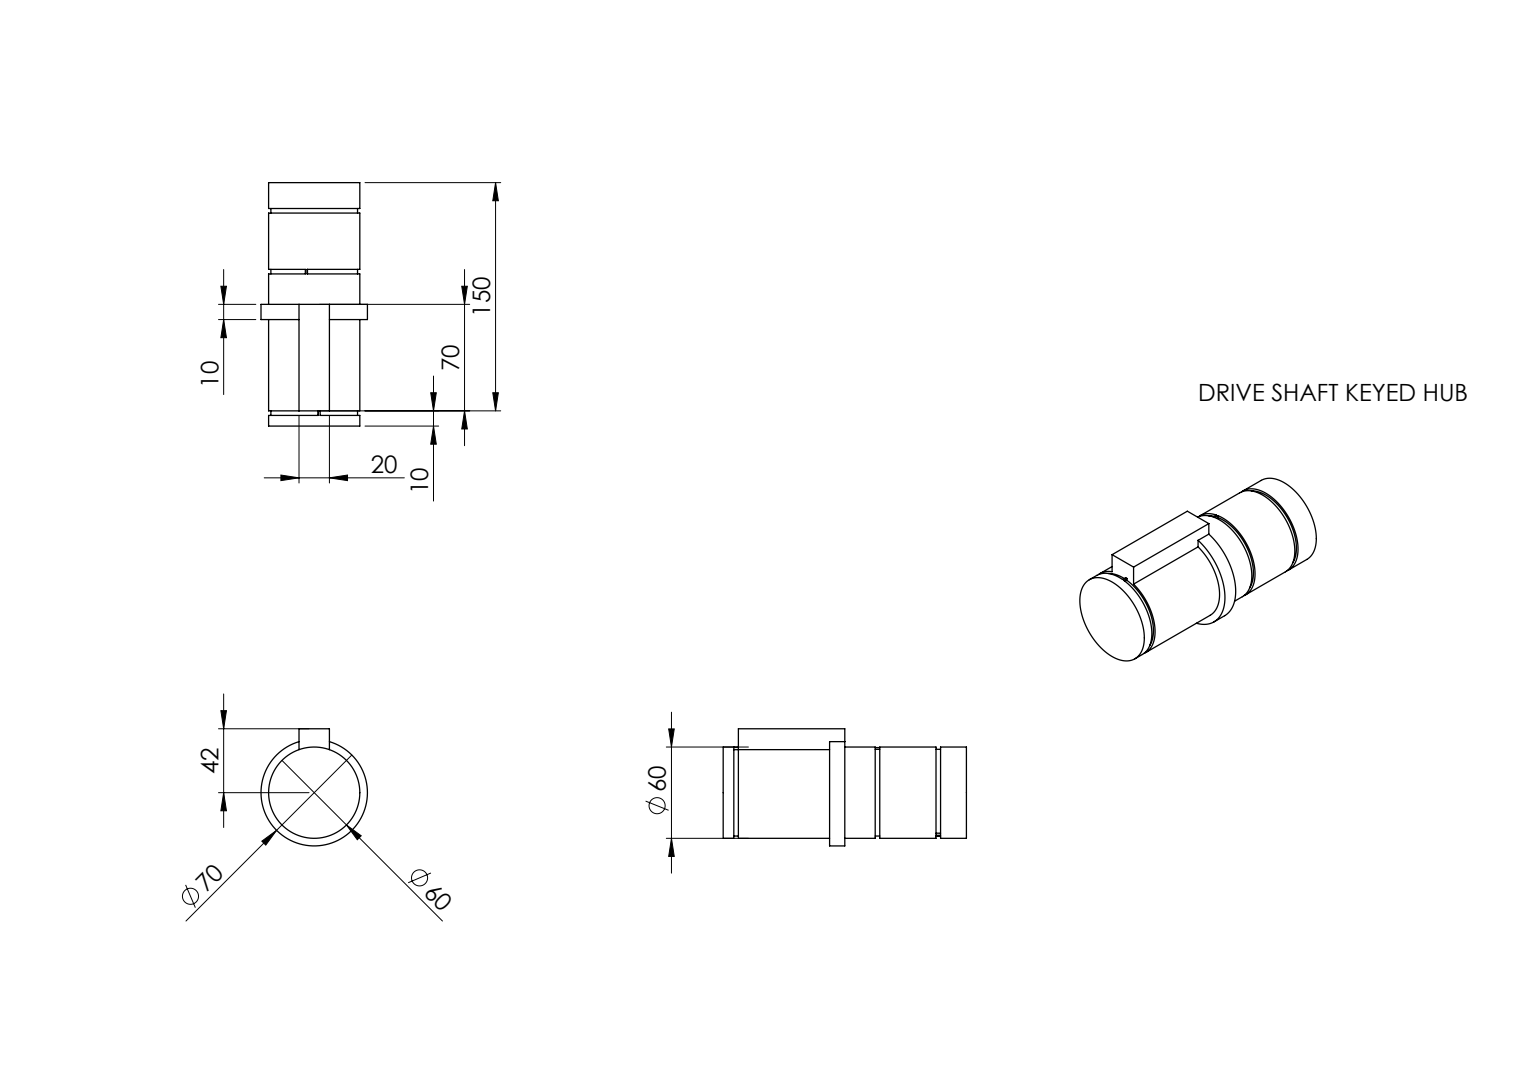
ISO-10303-21;
HEADER;
FILE_DESCRIPTION (('STEP AP214'),
    '1' );
FILE_NAME ('Drive Shaft Keyed Hub.step',
    '2026-10-23T05:12:30',
    ( '' ),
    ( '' ),
    'SwSTEP 2.0',
    'SolidWorks 2026',
    '' );
FILE_SCHEMA (( 'AUTOMOTIVE_DESIGN' ));
ENDSEC;

DATA;
#4=AXIS2_PLACEMENT_3D ( 'NONE', #5314, #2448, #2411 ) ;
#15=ORIENTED_EDGE ( 'NONE', *, *, #7014, .T. ) ;
#22=ORIENTED_EDGE ( 'NONE', *, *, #2120, .F. ) ;
#40=ADVANCED_FACE ( 'NONE', ( #3233 ), #3303, .T. ) ;
#41=ORIENTED_EDGE ( 'NONE', *, *, #4752, .T. ) ;
#44=LINE ( 'NONE', #2388, #7655 ) ;
#46=DIRECTION ( 'NONE',  ( 0.000000000000000000, -1.000000000000000000, 0.000000000000000000 ) ) ;
#47=VERTEX_POINT ( 'NONE', #965 ) ;
#48=EDGE_CURVE ( 'NONE', #5972, #47, #4560, .T. ) ;
#53=DIRECTION ( 'NONE',  ( 0.000000000000000000, 0.000000000000000000, -1.000000000000000000 ) ) ;
#68=LINE ( 'NONE', #4286, #4450 ) ;
#74=CARTESIAN_POINT ( 'NONE',  ( 9.568665290872617746, -28.43309066125681994, -139.9999999999999716 ) ) ;
#84=EDGE_CURVE ( 'NONE', #322, #6002, #3102, .T. ) ;
#89=EDGE_LOOP ( 'NONE', ( #7123, #2974, #1891, #2327 ) ) ;
#90=LINE ( 'NONE', #4231, #2988 ) ;
#97=ORIENTED_EDGE ( 'NONE', *, *, #4752, .F. ) ;
#103=LINE ( 'NONE', #1889, #2646 ) ;
#105=CIRCLE ( 'NONE', #7531, 28.50000000000000355 ) ;
#113=DIRECTION ( 'NONE',  ( 0.9412010056177179118, 0.3378471059875997051, 0.000000000000000000 ) ) ;
#116=ORIENTED_EDGE ( 'NONE', *, *, #4379, .T. ) ;
#118=ORIENTED_EDGE ( 'NONE', *, *, #897, .F. ) ;
#126=EDGE_LOOP ( 'NONE', ( #5453, #5673, #2876, #41 ) ) ;
#131=PRODUCT ( 'Drive Shaft Keyed Hub', 'Drive Shaft Keyed Hub', '', ( #3775 ) ) ;
#134=AXIS2_PLACEMENT_3D ( 'NONE', #2062, #2024, #2612 ) ;
#140=VECTOR ( 'NONE', #2880, 1000.000000000000000 ) ;
#149=ORIENTED_EDGE ( 'NONE', *, *, #2680, .T. ) ;
#150=DIRECTION ( 'NONE',  ( 0.9938725510941108787, -0.1105321318969463978, 0.000000000000000000 ) ) ;
#165=ORIENTED_EDGE ( 'NONE', *, *, #3978, .F. ) ;
#178=LINE ( 'NONE', #6692, #6392 ) ;
#180=STYLED_ITEM ( 'NONE', ( #6391 ), #5011 ) ;
#181=ADVANCED_FACE ( 'NONE', ( #7711 ), #4121, .F. ) ;
#188=ORIENTED_EDGE ( 'NONE', *, *, #6602, .F. ) ;
#194=VERTEX_POINT ( 'NONE', #3652 ) ;
#197=CARTESIAN_POINT ( 'NONE',  ( -5.554394503829287011, 27.95350964898380752, -79.99999999999995737 ) ) ;
#200=EDGE_LOOP ( 'NONE', ( #6714, #643, #5819, #2337 ) ) ;
#203=CARTESIAN_POINT ( 'NONE',  ( 9.090232026328989079, -27.01143612819398143, -119.9999999999999716 ) ) ;
#205=CARTESIAN_POINT ( 'NONE',  ( 9.090232026328989079, -27.01143612819398143, -122.9999999999999716 ) ) ;
#207=AXIS2_PLACEMENT_3D ( 'NONE', #2317, #4702, #7112 ) ;
#214=CARTESIAN_POINT ( 'NONE',  ( 5.777789833161707559E-31, -4.119912841284263785E-15, -119.9999999999999716 ) ) ;
#224=DIRECTION ( 'NONE',  ( 0.000000000000000000, 0.000000000000000000, -1.000000000000000000 ) ) ;
#226=CARTESIAN_POINT ( 'NONE',  ( -28.05900627794857627, -4.994213320838723824, -79.99999999999995737 ) ) ;
#228=DIRECTION ( 'NONE',  ( 0.000000000000000000, 0.000000000000000000, -1.000000000000000000 ) ) ;
#247=DIRECTION ( 'NONE',  ( -1.000000000000000000, 0.000000000000000000, 0.000000000000000000 ) ) ;
#249=DIRECTION ( 'NONE',  ( -0.09063257223759993431, -0.9958843993404034034, 0.000000000000000000 ) ) ;
#252=CYLINDRICAL_SURFACE ( 'NONE', #6988, 29.99999999999999289 ) ;
#256=VERTEX_POINT ( 'NONE', #1883 ) ;
#259=DIRECTION ( 'NONE',  ( -0.000000000000000000, -0.000000000000000000, 1.000000000000000000 ) ) ;
#264=ORIENTED_EDGE ( 'NONE', *, *, #3362, .F. ) ;
#266=ORIENTED_EDGE ( 'NONE', *, *, #6459, .F. ) ;
#267=CARTESIAN_POINT ( 'NONE',  ( 0.000000000000000000, 0.000000000000000000, -139.9999999999999716 ) ) ;
#270=CARTESIAN_POINT ( 'NONE',  ( 10.00000000000000000, 41.99999999999999289, -60.00000000000000711 ) ) ;
#279=FACE_OUTER_BOUND ( 'NONE', #4266, .T. ) ;
#281=ORIENTED_EDGE ( 'NONE', *, *, #3745, .T. ) ;
#284=CARTESIAN_POINT ( 'NONE',  ( 0.000000000000000000, 0.000000000000000000, -122.9999999999999716 ) ) ;
#287=CARTESIAN_POINT ( 'NONE',  ( 0.000000000000000000, 0.000000000000000000, -60.00000000000000000 ) ) ;
#292=EDGE_LOOP ( 'NONE', ( #3015, #4779, #3543, #2009 ) ) ;
#299=CARTESIAN_POINT ( 'NONE',  ( -10.00000000000000000, 28.28427124746189136, -50.00000000000000000 ) ) ;
#301=DIRECTION ( 'NONE',  ( 0.9412010056177179118, 0.3378471059875997051, 0.000000000000000000 ) ) ;
#303=VECTOR ( 'NONE', #4360, 1000.000000000000000 ) ;
#304=ORIENTED_EDGE ( 'NONE', *, *, #4363, .T. ) ;
#319=CIRCLE ( 'NONE', #5110, 29.99999999999999289 ) ;
#322=VERTEX_POINT ( 'NONE', #3771 ) ;
#333=ORIENTED_EDGE ( 'NONE', *, *, #3563, .F. ) ;
#341=CIRCLE ( 'NONE', #4254, 29.99999999999999289 ) ;
#344=ORIENTED_EDGE ( 'NONE', *, *, #1290, .F. ) ;
#349=CARTESIAN_POINT ( 'NONE',  ( 28.05900627794855851, 4.994213320838720271, -82.99999999999995737 ) ) ;
#353=CIRCLE ( 'NONE', #4261, 29.99999999999999289 ) ;
#368=DIRECTION ( 'NONE',  ( -1.000000000000000000, 0.000000000000000000, 0.000000000000000000 ) ) ;
#369=EDGE_CURVE ( 'NONE', #2537, #7447, #319, .T. ) ;
#382=AXIS2_PLACEMENT_3D ( 'NONE', #2843, #7643, #5876 ) ;
#383=ORIENTED_EDGE ( 'NONE', *, *, #6065, .F. ) ;
#385=DIRECTION ( 'NONE',  ( -1.000000000000000000, 0.000000000000000000, 0.000000000000000000 ) ) ;
#387=VERTEX_POINT ( 'NONE', #5026 ) ;
#394=EDGE_CURVE ( 'NONE', #2888, #7603, #5583, .T. ) ;
#398=DIRECTION ( 'NONE',  ( 1.000000000000000000, 0.000000000000000000, 0.000000000000000000 ) ) ;
#400=EDGE_CURVE ( 'NONE', #6073, #6532, #1763, .T. ) ;
#415=AXIS2_PLACEMENT_3D ( 'NONE', #6467, #428, #4730 ) ;
#427=FILL_AREA_STYLE ('',( #1657 ) ) ;
#428=DIRECTION ( 'NONE',  ( 3.081487911019577365E-33, -2.775557561562891967E-17, -1.000000000000000000 ) ) ;
#442=DIRECTION ( 'NONE',  ( 0.000000000000000000, 0.000000000000000000, 1.000000000000000000 ) ) ;
#443=DIRECTION ( 'NONE',  ( 1.000000000000000000, 0.000000000000000000, -0.000000000000000000 ) ) ;
#452=AXIS2_PLACEMENT_3D ( 'NONE', #5129, #1347, #6245 ) ;
#458=CARTESIAN_POINT ( 'NONE',  ( -6.873268260756527152E-15, 0.000000000000000000, -79.99999999999995737 ) ) ;
#459=ADVANCED_FACE ( 'NONE', ( #3218 ), #2157, .T. ) ;
#464=ORIENTED_EDGE ( 'NONE', *, *, #7412, .F. ) ;
#479=CARTESIAN_POINT ( 'NONE',  ( -7.039801714450301422E-15, 0.000000000000000000, -82.99999999999995737 ) ) ;
#480=AXIS2_PLACEMENT_3D ( 'NONE', #5844, #4103, #2188 ) ;
#481=DIRECTION ( 'NONE',  ( -0.000000000000000000, -0.000000000000000000, -1.000000000000000000 ) ) ;
#484=AXIS2_PLACEMENT_3D ( 'NONE', #5502, #2370, #2407 ) ;
#489=AXIS2_PLACEMENT_3D ( 'NONE', #1675, #1035, #3446 ) ;
#494=AXIS2_PLACEMENT_3D ( 'NONE', #1361, #3659, #3110 ) ;
#503=ORIENTED_EDGE ( 'NONE', *, *, #3907, .F. ) ;
#507=SURFACE_STYLE_FILL_AREA ( #427 ) ;
#512=EDGE_CURVE ( 'NONE', #3634, #5216, #2318, .T. ) ;
#518=CARTESIAN_POINT ( 'NONE',  ( 29.99999999999999289, 0.000000000000000000, -139.9999999999999716 ) ) ;
#526=FACE_OUTER_BOUND ( 'NONE', #5662, .T. ) ;
#531=VECTOR ( 'NONE', #6993, 1000.000000000000114 ) ;
#538=CYLINDRICAL_SURFACE ( 'NONE', #6515, 28.50000000000000711 ) ;
#542=AXIS2_PLACEMENT_3D ( 'NONE', #7456, #6279, #2065 ) ;
#558=EDGE_CURVE ( 'NONE', #1483, #3701, #583, .T. ) ;
#559=CARTESIAN_POINT ( 'NONE',  ( -10.00000000000000000, 28.28427124746189136, 10.00000000000000000 ) ) ;
#573=EDGE_CURVE ( 'NONE', #6864, #6819, #3734, .T. ) ;
#578=VERTEX_POINT ( 'NONE', #6013 ) ;
#583=CIRCLE ( 'NONE', #702, 29.99999999999999289 ) ;
#587=VERTEX_POINT ( 'NONE', #644 ) ;
#596=CARTESIAN_POINT ( 'NONE',  ( 0.000000000000000000, 0.000000000000000000, -79.99999999999995737 ) ) ;
#597=CYLINDRICAL_SURFACE ( 'NONE', #4258, 29.99999999999999289 ) ;
#599=VERTEX_POINT ( 'NONE', #3056 ) ;
#600=VECTOR ( 'NONE', #7039, 1000.000000000000000 ) ;
#613=ORIENTED_EDGE ( 'NONE', *, *, #2264, .T. ) ;
#617=AXIS2_PLACEMENT_3D ( 'NONE', #4825, #53, #3645 ) ;
#626=ORIENTED_EDGE ( 'NONE', *, *, #707, .F. ) ;
#628=ORIENTED_EDGE ( 'NONE', *, *, #2216, .T. ) ;
#629=CARTESIAN_POINT ( 'NONE',  ( -1.728922298134113098E-15, 8.513302795252935035E-16, 10.00000000000000000 ) ) ;
#635=ORIENTED_EDGE ( 'NONE', *, *, #878, .T. ) ;
#636=AXIS2_PLACEMENT_3D ( 'NONE', #596, #7064, #5883 ) ;
#643=ORIENTED_EDGE ( 'NONE', *, *, #5237, .F. ) ;
#644=CARTESIAN_POINT ( 'NONE',  ( 29.99999999999999289, 0.000000000000000000, -60.00000000000000000 ) ) ;
#667=LINE ( 'NONE', #5442, #3443 ) ;
#672=EDGE_CURVE ( 'NONE', #3192, #3615, #90, .T. ) ;
#681=VECTOR ( 'NONE', #5176, 1000.000000000000000 ) ;
#682=CARTESIAN_POINT ( 'NONE',  ( 3.716043017018883621, 28.25669875083898930, 13.00000000000000178 ) ) ;
#683=CARTESIAN_POINT ( 'NONE',  ( -26.82422866010495710, -9.628642520646591763, -122.9999999999999716 ) ) ;
#692=DIRECTION ( 'NONE',  ( 0.000000000000000000, 0.000000000000000000, 1.000000000000000000 ) ) ;
#700=ADVANCED_FACE ( 'NONE', ( #3679 ), #2979, .T. ) ;
#702=AXIS2_PLACEMENT_3D ( 'NONE', #2238, #7036, #2274 ) ;
#706=DIRECTION ( 'NONE',  ( -0.000000000000000000, 1.000000000000000000, 0.000000000000000000 ) ) ;
#707=EDGE_CURVE ( 'NONE', #2049, #6833, #1270, .T. ) ;
#709=CIRCLE ( 'NONE', #6257, 28.50000000000000711 ) ;
#711=CYLINDRICAL_SURFACE ( 'NONE', #6817, 29.99999999999999289 ) ;
#726=ORIENTED_EDGE ( 'NONE', *, *, #6984, .F. ) ;
#750=DIRECTION ( 'NONE',  ( 0.000000000000000000, 0.000000000000000000, 1.000000000000000000 ) ) ;
#751=FACE_OUTER_BOUND ( 'NONE', #3367, .T. ) ;
#757=EDGE_CURVE ( 'NONE', #3192, #1710, #4102, .T. ) ;
#770=DIRECTION ( 'NONE',  ( -0.1555099737793451398, 0.9878343221690302212, -1.110223024625155986E-18 ) ) ;
#775=EDGE_LOOP ( 'NONE', ( #5683, #7161, #971, #2534, #5294, #5753, #1571, #266 ) ) ;
#778=CARTESIAN_POINT ( 'NONE',  ( -7.039801714450301422E-15, 0.000000000000000000, -82.99999999999995737 ) ) ;
#779=AXIS2_PLACEMENT_3D ( 'NONE', #837, #6286, #2075 ) ;
#783=PRODUCT_DEFINITION_FORMATION_WITH_SPECIFIED_SOURCE ( 'ANY', '', #131, .NOT_KNOWN. ) ;
#792=VECTOR ( 'NONE', #1139, 1000.000000000000000 ) ;
#804=FACE_OUTER_BOUND ( 'NONE', #126, .T. ) ;
#811=ORIENTED_EDGE ( 'NONE', *, *, #4867, .T. ) ;
#823=AXIS2_PLACEMENT_3D ( 'NONE', #1004, #3418, #6495 ) ;
#837=CARTESIAN_POINT ( 'NONE',  ( -1.728922298134113098E-15, 8.513302795252935035E-16, 13.00000000000000178 ) ) ;
#841=DIRECTION ( 'NONE',  ( 0.000000000000000000, -1.000000000000000000, 0.000000000000000000 ) ) ;
#842=VECTOR ( 'NONE', #3621, 1000.000000000000000 ) ;
#845=DIRECTION ( 'NONE',  ( -0.000000000000000000, -0.000000000000000000, 1.000000000000000000 ) ) ;
#859=VECTOR ( 'NONE', #5866, 1000.000000000000000 ) ;
#861=DIRECTION ( 'NONE',  ( 1.000000000000000000, 0.000000000000000000, -0.000000000000000000 ) ) ;
#865=CARTESIAN_POINT ( 'NONE',  ( -6.873268260756527152E-15, 0.000000000000000000, -79.99999999999995737 ) ) ;
#866=DIRECTION ( 'NONE',  ( 0.000000000000000000, 0.000000000000000000, -1.000000000000000000 ) ) ;
#876=CARTESIAN_POINT ( 'NONE',  ( 0.000000000000000000, 0.000000000000000000, -50.00000000000000000 ) ) ;
#878=EDGE_CURVE ( 'NONE', #5239, #4532, #709, .T. ) ;
#882=DIRECTION ( 'NONE',  ( 0.000000000000000000, 0.000000000000000000, 1.000000000000000000 ) ) ;
#883=AXIS2_PLACEMENT_3D ( 'NONE', #1655, #1745, #6464 ) ;
#886=VERTEX_POINT ( 'NONE', #1504 ) ;
#897=EDGE_CURVE ( 'NONE', #5940, #2183, #5745, .T. ) ;
#911=VECTOR ( 'NONE', #4475, 1000.000000000000000 ) ;
#915=CARTESIAN_POINT ( 'NONE',  ( 28.05900627794856206, 4.994213320838721160, -79.99999999999995737 ) ) ;
#916=AXIS2_PLACEMENT_3D ( 'NONE', #6341, #927, #3343 ) ;
#921=DIRECTION ( 'NONE',  ( 3.081487911019577365E-33, -2.775557561562891967E-17, -1.000000000000000000 ) ) ;
#927=DIRECTION ( 'NONE',  ( 0.000000000000000000, 0.000000000000000000, 1.000000000000000000 ) ) ;
#928=VECTOR ( 'NONE', #3765, 1000.000000000000114 ) ;
#929=DIRECTION ( 'NONE',  ( 0.3566035499204626702, -0.9342558044690565389, 2.649161120199466423E-17 ) ) ;
#939=CARTESIAN_POINT ( 'NONE',  ( 29.99999999999999289, 0.000000000000000000, -139.9999999999999716 ) ) ;
#948=CARTESIAN_POINT ( 'NONE',  ( -29.99999999999999289, 3.673940397442058389E-15, -122.9999999999999716 ) ) ;
#950=CARTESIAN_POINT ( 'NONE',  ( -4.665299213380365018, 29.63502966507090619, -139.9999999999999716 ) ) ;
#952=VERTEX_POINT ( 'NONE', #1020 ) ;
#960=DIRECTION ( 'NONE',  ( 5.551115123125782702E-17, 0.000000000000000000, 1.000000000000000000 ) ) ;
#965=CARTESIAN_POINT ( 'NONE',  ( -4.432034252711344102, 28.15327818181735964, -82.99999999999995737 ) ) ;
#971=ORIENTED_EDGE ( 'NONE', *, *, #5971, .T. ) ;
#972=ORIENTED_EDGE ( 'NONE', *, *, #2975, .F. ) ;
#973=ORIENTED_EDGE ( 'NONE', *, *, #1738, .F. ) ;
#981=AXIS2_PLACEMENT_3D ( 'NONE', #197, #6831, #1415 ) ;
#1003=EDGE_CURVE ( 'NONE', #3123, #7368, #6511, .T. ) ;
#1004=CARTESIAN_POINT ( 'NONE',  ( -1.728922298134113098E-15, 8.513302795252935035E-16, 13.00000000000000178 ) ) ;
#1008=CIRCLE ( 'NONE', #134, 29.99999999999999289 ) ;
#1013=AXIS2_PLACEMENT_3D ( 'NONE', #629, #4330, #150 ) ;
#1016=( NAMED_UNIT ( * ) PLANE_ANGLE_UNIT ( ) SI_UNIT ( $, .RADIAN. ) );
#1020=CARTESIAN_POINT ( 'NONE',  ( -5.554394503829287011, 27.95350964898380752, -79.99999999999995737 ) ) ;
#1027=EDGE_CURVE ( 'NONE', #5335, #5921, #6769, .T. ) ;
#1030=ADVANCED_FACE ( 'NONE', ( #7613 ), #2230, .F. ) ;
#1035=DIRECTION ( 'NONE',  ( 0.9958843993404035144, -0.09063257223759993431, 0.000000000000000000 ) ) ;
#1039=CARTESIAN_POINT ( 'NONE',  ( -4.432034252711344102, 28.15327818181735964, -79.99999999999995737 ) ) ;
#1043=VERTEX_POINT ( 'NONE', #5371 ) ;
#1044=ADVANCED_FACE ( 'NONE', ( #1431 ), #3848, .F. ) ;
#1047=DIRECTION ( 'NONE',  ( -3.081487911019577365E-33, 2.775557561562891967E-17, 1.000000000000000000 ) ) ;
#1049=VECTOR ( 'NONE', #6193, 1000.000000000000000 ) ;
#1051=VERTEX_POINT ( 'NONE', #6214 ) ;
#1057=CARTESIAN_POINT ( 'NONE',  ( 10.16320117273318679, -26.62629042736811869, -122.9999999999999716 ) ) ;
#1059=SURFACE_SIDE_STYLE ('',( #507 ) ) ;
#1061=AXIS2_PLACEMENT_3D ( 'NONE', #6484, #7155, #7343 ) ;
#1076=CARTESIAN_POINT ( 'NONE',  ( -10.00000000000000000, 0.000000000000000000, -60.00000000000000711 ) ) ;
#1084=EDGE_CURVE ( 'NONE', #2183, #6897, #6251, .T. ) ;
#1098=CIRCLE ( 'NONE', #5510, 29.99999999999999289 ) ;
#1102=VERTEX_POINT ( 'NONE', #6177 ) ;
#1105=DIRECTION ( 'NONE',  ( 0.9412010056177179118, 0.3378471059875997051, 0.000000000000000000 ) ) ;
#1106=CARTESIAN_POINT ( 'NONE',  ( -6.873268260756527152E-15, 0.000000000000000000, -79.99999999999995737 ) ) ;
#1108=CARTESIAN_POINT ( 'NONE',  ( -29.99999999999999289, 3.673940397442058389E-15, 10.00000000000000888 ) ) ;
#1119=CARTESIAN_POINT ( 'NONE',  ( -28.05900627794857272, -4.994213320838722936, -79.99999999999995737 ) ) ;
#1124=CARTESIAN_POINT ( 'NONE',  ( -7.039801714450301422E-15, 0.000000000000000000, -82.99999999999995737 ) ) ;
#1126=LINE ( 'NONE', #4642, #3627 ) ;
#1134=AXIS2_PLACEMENT_3D ( 'NONE', #4260, #7227, #1827 ) ;
#1139=DIRECTION ( 'NONE',  ( -0.1555099737793451675, 0.9878343221690302212, -1.110223024625155986E-18 ) ) ;
#1140=EDGE_CURVE ( 'NONE', #4191, #4160, #4986, .T. ) ;
#1146=DIRECTION ( 'NONE',  ( 0.9845265360683707057, 0.1752355551171480841, 0.000000000000000000 ) ) ;
#1147=DIRECTION ( 'NONE',  ( 0.000000000000000000, 0.000000000000000000, 1.000000000000000000 ) ) ;
#1162=CIRCLE ( 'NONE', #3063, 29.99999999999999289 ) ;
#1173=EDGE_LOOP ( 'NONE', ( #97, #3739, #149, #5750, #3439, #1470 ) ) ;
#1179=MECHANICAL_DESIGN_GEOMETRIC_PRESENTATION_REPRESENTATION('',(#3832),#5212);
#1199=LINE ( 'NONE', #4350, #6780 ) ;
#1205=LINE ( 'NONE', #3620, #3011 ) ;
#1206=DIRECTION ( 'NONE',  ( 0.000000000000000000, 0.000000000000000000, -1.000000000000000000 ) ) ;
#1217=LINE ( 'NONE', #4845, #1423 ) ;
#1224=FACE_OUTER_BOUND ( 'NONE', #5370, .T. ) ;
#1232=CARTESIAN_POINT ( 'NONE',  ( 0.000000000000000000, 0.000000000000000000, -139.9999999999999716 ) ) ;
#1248=CARTESIAN_POINT ( 'NONE',  ( 10.00000000000000000, 28.28427124746189136, 10.00000000000000888 ) ) ;
#1258=CARTESIAN_POINT ( 'NONE',  ( -29.99999999999999289, 3.673940397442058389E-15, 13.00000000000001066 ) ) ;
#1267=ORIENTED_EDGE ( 'NONE', *, *, #5379, .T. ) ;
#1270=LINE ( 'NONE', #682, #7760 ) ;
#1282=LINE ( 'NONE', #3774, #4249 ) ;
#1287=ORIENTED_EDGE ( 'NONE', *, *, #1958, .T. ) ;
#1290=EDGE_CURVE ( 'NONE', #6532, #7160, #3619, .T. ) ;
#1300=DIRECTION ( 'NONE',  ( 1.000000000000000000, 0.000000000000000000, 0.000000000000000000 ) ) ;
#1301=CARTESIAN_POINT ( 'NONE',  ( 0.000000000000000000, 0.000000000000000000, 0.000000000000000000 ) ) ;
#1306=ORIENTED_EDGE ( 'NONE', *, *, #5427, .F. ) ;
#1310=DIRECTION ( 'NONE',  ( -1.000000000000000000, -8.881784197001252323E-16, 0.000000000000000000 ) ) ;
#1315=AXIS2_PLACEMENT_3D ( 'NONE', #7626, #4670, #6374 ) ;
#1318=DIRECTION ( 'NONE',  ( 0.1303874742813643239, 0.9914631140645255858, 0.000000000000000000 ) ) ;
#1324=DIRECTION ( 'NONE',  ( 0.000000000000000000, 0.000000000000000000, -1.000000000000000000 ) ) ;
#1325=VERTEX_POINT ( 'NONE', #3442 ) ;
#1331=DIRECTION ( 'NONE',  ( 3.081487911019577365E-33, -2.775557561562891967E-17, -1.000000000000000000 ) ) ;
#1332=CYLINDRICAL_SURFACE ( 'NONE', #6222, 28.50000000000000711 ) ;
#1346=ORIENTED_EDGE ( 'NONE', *, *, #4608, .F. ) ;
#1347=DIRECTION ( 'NONE',  ( 5.551115123125782702E-17, -0.000000000000000000, 1.000000000000000000 ) ) ;
#1357=DIRECTION ( 'NONE',  ( -0.000000000000000000, -0.000000000000000000, 1.000000000000000000 ) ) ;
#1361=CARTESIAN_POINT ( 'NONE',  ( 0.000000000000000000, 0.000000000000000000, -60.00000000000000711 ) ) ;
#1362=ORIENTED_EDGE ( 'NONE', *, *, #1084, .F. ) ;
#1363=EDGE_LOOP ( 'NONE', ( #383, #2492 ) ) ;
#1368=CARTESIAN_POINT ( 'NONE',  ( 5.870234470492294880E-31, -4.203179568131150526E-15, -122.9999999999999716 ) ) ;
#1371=ORIENTED_EDGE ( 'NONE', *, *, #1525, .F. ) ;
#1377=EDGE_CURVE ( 'NONE', #1051, #6864, #5904, .T. ) ;
#1382=CARTESIAN_POINT ( 'NONE',  ( 3.911624228440929052, 29.74389342193576624, 13.00000000000001066 ) ) ;
#1383=ORIENTED_EDGE ( 'NONE', *, *, #3503, .F. ) ;
#1387=PRODUCT_DEFINITION_SHAPE ( 'NONE', 'NONE',  #6478 ) ;
#1392=LINE ( 'NONE', #205, #6581 ) ;
#1393=ORIENTED_EDGE ( 'NONE', *, *, #6504, .T. ) ;
#1409=EDGE_LOOP ( 'NONE', ( #1796, #3155, #6670, #4098, #6477, #628 ) ) ;
#1413=DIRECTION ( 'NONE',  ( 0.9845265360683707057, 0.1752355551171480841, 0.000000000000000000 ) ) ;
#1415=DIRECTION ( 'NONE',  ( 0.1948910352220799835, -0.9808248999643441879, -1.110223024625155986E-18 ) ) ;
#1423=VECTOR ( 'NONE', #706, 1000.000000000000000 ) ;
#1431=FACE_OUTER_BOUND ( 'NONE', #2465, .T. ) ;
#1443=EDGE_CURVE ( 'NONE', #7492, #5665, #1126, .T. ) ;
#1446=CLOSED_SHELL ( 'NONE', ( #6737, #6352, #1475, #5330, #3466, #2829, #4656, #459, #3800, #2519, #2309, #7588, #4374, #5871, #7324, #3599, #2557, #7263, #7513, #700, #4765, #1030, #2895, #40, #4909, #3685, #2653, #2637, #1589, #5674, #181, #5443, #6790, #5617, #2777, #1044, #5963, #4858, #7757, #1575 ) ) ;
#1465=AXIS2_PLACEMENT_3D ( 'NONE', #1909, #5531, #2395 ) ;
#1470=ORIENTED_EDGE ( 'NONE', *, *, #7693, .T. ) ;
#1475=ADVANCED_FACE ( 'NONE', ( #3538 ), #538, .T. ) ;
#1481=DIRECTION ( 'NONE',  ( 3.081487911019577365E-33, -2.775557561562891967E-17, -1.000000000000000000 ) ) ;
#1482=EDGE_LOOP ( 'NONE', ( #6953, #7658, #5675, #1661, #7308, #6188, #4056, #2700 ) ) ;
#1483=VERTEX_POINT ( 'NONE', #2371 ) ;
#1486=EDGE_CURVE ( 'NONE', #7492, #2049, #3874, .T. ) ;
#1495=ORIENTED_EDGE ( 'NONE', *, *, #7454, .F. ) ;
#1497=DIRECTION ( 'NONE',  ( 0.000000000000000000, 0.000000000000000000, 1.000000000000000000 ) ) ;
#1504=CARTESIAN_POINT ( 'NONE',  ( -28.32536770618215982, 3.150165759062969695, 10.00000000000000000 ) ) ;
#1505=CARTESIAN_POINT ( 'NONE',  ( 28.32536770618215982, -3.150165759062971471, 13.00000000000000178 ) ) ;
#1507=AXIS2_PLACEMENT_3D ( 'NONE', #6309, #7594, #7009 ) ;
#1511=AXIS2_PLACEMENT_3D ( 'NONE', #5290, #6517, #6472 ) ;
#1519=VECTOR ( 'NONE', #1931, 1000.000000000000000 ) ;
#1521=ORIENTED_EDGE ( 'NONE', *, *, #7357, .F. ) ;
#1522=EDGE_CURVE ( 'NONE', #2129, #7160, #1282, .T. ) ;
#1525=EDGE_CURVE ( 'NONE', #4724, #194, #4873, .T. ) ;
#1545=DIRECTION ( 'NONE',  ( 1.000000000000000000, 0.000000000000000000, 0.000000000000000000 ) ) ;
#1552=CARTESIAN_POINT ( 'NONE',  ( -4.665299213380359689, 29.63502966507089909, -79.99999999999995737 ) ) ;
#1553=PLANE ( 'NONE',  #489 ) ;
#1559=VECTOR ( 'NONE', #6445, 1000.000000000000000 ) ;
#1562=DIRECTION ( 'NONE',  ( -5.551115123125782702E-17, 0.000000000000000000, -1.000000000000000000 ) ) ;
#1564=COLOUR_RGB ( '',0.8941176470588234615, 0.8941176470588234615, 0.8941176470588234615 ) ;
#1571=ORIENTED_EDGE ( 'NONE', *, *, #5379, .F. ) ;
#1573=VERTEX_POINT ( 'NONE', #4989 ) ;
#1575=ADVANCED_FACE ( 'NONE', ( #4243 ), #3067, .T. ) ;
#1588=LINE ( 'NONE', #5293, #531 ) ;
#1589=ADVANCED_FACE ( 'NONE', ( #4357 ), #3691, .F. ) ;
#1591=AXIS2_PLACEMENT_3D ( 'NONE', #7063, #5328, #7728 ) ;
#1596=CARTESIAN_POINT ( 'NONE',  ( 29.99999999999999289, 0.000000000000000000, -139.9999999999999716 ) ) ;
#1601=VERTEX_POINT ( 'NONE', #2597 ) ;
#1616=DIRECTION ( 'NONE',  ( 0.000000000000000000, 0.000000000000000000, 1.000000000000000000 ) ) ;
#1619=EDGE_CURVE ( 'NONE', #3881, #2383, #178, .T. ) ;
#1627=ORIENTED_EDGE ( 'NONE', *, *, #5133, .F. ) ;
#1635=FACE_OUTER_BOUND ( 'NONE', #3761, .T. ) ;
#1654=AXIS2_PLACEMENT_3D ( 'NONE', #1124, #2331, #5941 ) ;
#1655=CARTESIAN_POINT ( 'NONE',  ( -1.728922298134113098E-15, 8.513302795252935035E-16, 13.00000000000000178 ) ) ;
#1657=FILL_AREA_STYLE_COLOUR ( '', #1564 ) ;
#1658=FACE_OUTER_BOUND ( 'NONE', #6506, .T. ) ;
#1661=ORIENTED_EDGE ( 'NONE', *, *, #5964, .T. ) ;
#1672=CIRCLE ( 'NONE', #5195, 29.99999999999999289 ) ;
#1675=CARTESIAN_POINT ( 'NONE',  ( 2.583028308771596837, 28.38270538120150377, 13.00000000000000178 ) ) ;
#1679=ORIENTED_EDGE ( 'NONE', *, *, #2459, .F. ) ;
#1689=CARTESIAN_POINT ( 'NONE',  ( 26.82422866010495710, 9.628642520646586433, -119.9999999999999716 ) ) ;
#1691=EDGE_CURVE ( 'NONE', #6167, #587, #1098, .T. ) ;
#1693=EDGE_LOOP ( 'NONE', ( #1306, #6106, #1845, #1679, #5241, #2719 ) ) ;
#1710=VERTEX_POINT ( 'NONE', #2668 ) ;
#1716=DIRECTION ( 'NONE',  ( 1.000000000000000000, 0.000000000000000000, 0.000000000000000000 ) ) ;
#1727=EDGE_CURVE ( 'NONE', #194, #5633, #2123, .T. ) ;
#1738=EDGE_CURVE ( 'NONE', #1573, #322, #3257, .T. ) ;
#1745=DIRECTION ( 'NONE',  ( 0.000000000000000000, 0.000000000000000000, 1.000000000000000000 ) ) ;
#1754=CYLINDRICAL_SURFACE ( 'NONE', #5016, 29.99999999999999289 ) ;
#1763=LINE ( 'NONE', #5342, #6614 ) ;
#1765=LINE ( 'NONE', #2398, #5008 ) ;
#1767=CARTESIAN_POINT ( 'NONE',  ( -29.99999999999999289, 3.673940397442058389E-15, -139.9999999999999716 ) ) ;
#1791=ORIENTED_EDGE ( 'NONE', *, *, #84, .F. ) ;
#1794=DIRECTION ( 'NONE',  ( -0.000000000000000000, -0.000000000000000000, 1.000000000000000000 ) ) ;
#1796=ORIENTED_EDGE ( 'NONE', *, *, #7701, .T. ) ;
#1806=AXIS2_PLACEMENT_3D ( 'NONE', #7147, #3053, #3558 ) ;
#1821=DIRECTION ( 'NONE',  ( 0.9845265360683707057, 0.1752355551171480841, 0.000000000000000000 ) ) ;
#1827=DIRECTION ( 'NONE',  ( 0.9938725510941108787, -0.1105321318969463978, 0.000000000000000000 ) ) ;
#1833=ORIENTED_EDGE ( 'NONE', *, *, #400, .F. ) ;
#1845=ORIENTED_EDGE ( 'NONE', *, *, #1140, .F. ) ;
#1848=DIRECTION ( 'NONE',  ( 0.9938725510941107677, -0.1105321318969463978, 0.000000000000000000 ) ) ;
#1871=EDGE_CURVE ( 'NONE', #3192, #952, #1765, .T. ) ;
#1874=DIRECTION ( 'NONE',  ( 1.000000000000000000, 0.000000000000000000, 0.000000000000000000 ) ) ;
#1879=DIRECTION ( 'NONE',  ( 0.000000000000000000, 0.000000000000000000, 1.000000000000000000 ) ) ;
#1883=CARTESIAN_POINT ( 'NONE',  ( 10.00000000000000000, 33.54101966249685773, -60.00000000000000711 ) ) ;
#1889=CARTESIAN_POINT ( 'NONE',  ( -29.99999999999999289, 3.673940397442058389E-15, -139.9999999999999716 ) ) ;
#1891=ORIENTED_EDGE ( 'NONE', *, *, #394, .F. ) ;
#1892=EDGE_LOOP ( 'NONE', ( #7570, #7268, #5159, #7586 ) ) ;
#1897=DIRECTION ( 'NONE',  ( -3.081487911019577365E-33, 2.775557561562891967E-17, 1.000000000000000000 ) ) ;
#1901=CIRCLE ( 'NONE', #6681, 35.00000000000000711 ) ;
#1903=CARTESIAN_POINT ( 'NONE',  ( 9.568665290872615969, -28.43309066125680928, -122.9999999999999716 ) ) ;
#1909=CARTESIAN_POINT ( 'NONE',  ( 0.000000000000000000, 0.000000000000000000, -82.99999999999995737 ) ) ;
#1915=DIRECTION ( 'NONE',  ( 1.000000000000000000, 0.000000000000000000, 0.000000000000000000 ) ) ;
#1928=ORIENTED_EDGE ( 'NONE', *, *, #1486, .F. ) ;
#1931=DIRECTION ( 'NONE',  ( 0.000000000000000000, 0.000000000000000000, 1.000000000000000000 ) ) ;
#1938=EDGE_LOOP ( 'NONE', ( #464, #4811, #3806, #503, #3845, #333 ) ) ;
#1958=EDGE_CURVE ( 'NONE', #4364, #7642, #341, .T. ) ;
#1964=DIRECTION ( 'NONE',  ( 0.000000000000000000, 0.000000000000000000, -1.000000000000000000 ) ) ;
#1968=EDGE_CURVE ( 'NONE', #3701, #2140, #7000, .T. ) ;
#1972=VERTEX_POINT ( 'NONE', #7276 ) ;
#2002=CARTESIAN_POINT ( 'NONE',  ( 10.69810649761387822, -28.02767413407169528, -122.9999999999999716 ) ) ;
#2009=ORIENTED_EDGE ( 'NONE', *, *, #1619, .T. ) ;
#2013=ORIENTED_EDGE ( 'NONE', *, *, #2459, .T. ) ;
#2021=ORIENTED_EDGE ( 'NONE', *, *, #6504, .F. ) ;
#2022=ORIENTED_EDGE ( 'NONE', *, *, #2069, .F. ) ;
#2024=DIRECTION ( 'NONE',  ( -0.000000000000000000, -0.000000000000000000, 1.000000000000000000 ) ) ;
#2030=AXIS2_PLACEMENT_3D ( 'NONE', #6230, #1331, #7296 ) ;
#2032=CARTESIAN_POINT ( 'NONE',  ( 5.870234470492294880E-31, -4.203179568131150526E-15, -122.9999999999999716 ) ) ;
#2033=CARTESIAN_POINT ( 'NONE',  ( 0.000000000000000000, 0.000000000000000000, -50.00000000000000000 ) ) ;
#2036=CYLINDRICAL_SURFACE ( 'NONE', #779, 28.50000000000000711 ) ;
#2046=DIRECTION ( 'NONE',  ( 1.000000000000000000, 0.000000000000000000, 0.000000000000000000 ) ) ;
#2048=ORIENTED_EDGE ( 'NONE', *, *, #5769, .T. ) ;
#2049=VERTEX_POINT ( 'NONE', #3021 ) ;
#2052=ORIENTED_EDGE ( 'NONE', *, *, #5481, .F. ) ;
#2062=CARTESIAN_POINT ( 'NONE',  ( 0.000000000000000000, 0.000000000000000000, 13.00000000000001066 ) ) ;
#2064=FACE_OUTER_BOUND ( 'NONE', #6156, .T. ) ;
#2065=DIRECTION ( 'NONE',  ( -0.3189555096957539804, 0.9477696887085605981, -2.581026109104742394E-17 ) ) ;
#2069=EDGE_CURVE ( 'NONE', #1601, #6833, #1199, .T. ) ;
#2071=DIRECTION ( 'NONE',  ( 0.000000000000000000, 0.000000000000000000, 1.000000000000000000 ) ) ;
#2075=DIRECTION ( 'NONE',  ( 0.9938725510941108787, -0.1105321318969463978, 0.000000000000000000 ) ) ;
#2078=AXIS2_PLACEMENT_3D ( 'NONE', #4306, #6717, #1310 ) ;
#2085=AXIS2_PLACEMENT_3D ( 'NONE', #7746, #3413, #6449 ) ;
#2088=VERTEX_POINT ( 'NONE', #5424 ) ;
#2104=DIRECTION ( 'NONE',  ( 1.000000000000000000, 0.000000000000000000, 0.000000000000000000 ) ) ;
#2116=EDGE_CURVE ( 'NONE', #2383, #5846, #6206, .T. ) ;
#2120=EDGE_CURVE ( 'NONE', #5661, #3942, #2739, .T. ) ;
#2123=CIRCLE ( 'NONE', #7514, 35.00000000000000711 ) ;
#2129=VERTEX_POINT ( 'NONE', #3804 ) ;
#2138=ORIENTED_EDGE ( 'NONE', *, *, #6395, .F. ) ;
#2140=VERTEX_POINT ( 'NONE', #5725 ) ;
#2142=FACE_OUTER_BOUND ( 'NONE', #2574, .T. ) ;
#2157=CYLINDRICAL_SURFACE ( 'NONE', #6876, 35.00000000000000711 ) ;
#2171=LINE ( 'NONE', #7085, #3144 ) ;
#2183=VERTEX_POINT ( 'NONE', #4503 ) ;
#2184=VECTOR ( 'NONE', #5450, 1000.000000000000000 ) ;
#2188=DIRECTION ( 'NONE',  ( 0.9845265360683707057, 0.1752355551171480841, 0.000000000000000000 ) ) ;
#2201=VERTEX_POINT ( 'NONE', #203 ) ;
#2204=ORIENTED_EDGE ( 'NONE', *, *, #3180, .F. ) ;
#2209=EDGE_CURVE ( 'NONE', #7320, #7642, #3211, .T. ) ;
#2214=DIRECTION ( 'NONE',  ( 0.000000000000000000, 0.000000000000000000, 1.000000000000000000 ) ) ;
#2216=EDGE_CURVE ( 'NONE', #7160, #2888, #7407, .T. ) ;
#2230=PLANE ( 'NONE',  #5632 ) ;
#2238=CARTESIAN_POINT ( 'NONE',  ( 0.000000000000000000, 0.000000000000000000, -139.9999999999999716 ) ) ;
#2243=CARTESIAN_POINT ( 'NONE',  ( -28.32536770618215982, 3.150165759062969695, 13.00000000000000178 ) ) ;
#2253=DIRECTION ( 'NONE',  ( 1.000000000000000000, 0.000000000000000000, 0.000000000000000000 ) ) ;
#2264=EDGE_CURVE ( 'NONE', #4532, #4648, #7654, .T. ) ;
#2266=DIRECTION ( 'NONE',  ( -1.000000000000000000, 0.000000000000000000, 0.000000000000000000 ) ) ;
#2267=DIRECTION ( 'NONE',  ( -1.000000000000000000, 0.000000000000000000, 0.000000000000000000 ) ) ;
#2274=DIRECTION ( 'NONE',  ( 1.000000000000000000, 0.000000000000000000, 0.000000000000000000 ) ) ;
#2276=CARTESIAN_POINT ( 'NONE',  ( 29.99999999999999289, 0.000000000000000000, -139.9999999999999716 ) ) ;
#2277=LINE ( 'NONE', #2783, #4141 ) ;
#2284=CIRCLE ( 'NONE', #5292, 28.50000000000000355 ) ;
#2300=( NAMED_UNIT ( * ) SI_UNIT ( $, .STERADIAN. ) SOLID_ANGLE_UNIT ( ) );
#2303=CARTESIAN_POINT ( 'NONE',  ( -29.99999999999999289, 3.673940397442058389E-15, -82.99999999999995737 ) ) ;
#2309=ADVANCED_FACE ( 'NONE', ( #6475 ), #1754, .T. ) ;
#2317=CARTESIAN_POINT ( 'NONE',  ( 0.000000000000000000, 0.000000000000000000, 10.00000000000000888 ) ) ;
#2318=LINE ( 'NONE', #6410, #2488 ) ;
#2326=ORIENTED_EDGE ( 'NONE', *, *, #84, .T. ) ;
#2327=ORIENTED_EDGE ( 'NONE', *, *, #2216, .F. ) ;
#2331=DIRECTION ( 'NONE',  ( -5.635681009894454322E-17, -1.505185443864239327E-19, -1.000000000000000000 ) ) ;
#2337=ORIENTED_EDGE ( 'NONE', *, *, #4723, .T. ) ;
#2340=ORIENTED_EDGE ( 'NONE', *, *, #1003, .F. ) ;
#2357=EDGE_CURVE ( 'NONE', #952, #5940, #6912, .T. ) ;
#2361=CARTESIAN_POINT ( 'NONE',  ( 0.000000000000000000, 0.000000000000000000, -79.99999999999995737 ) ) ;
#2366=ORIENTED_EDGE ( 'NONE', *, *, #5394, .T. ) ;
#2368=EDGE_CURVE ( 'NONE', #6897, #47, #105, .T. ) ;
#2370=DIRECTION ( 'NONE',  ( 0.000000000000000000, 0.000000000000000000, -1.000000000000000000 ) ) ;
#2371=CARTESIAN_POINT ( 'NONE',  ( -29.99999999999999289, 3.673940397442058389E-15, -139.9999999999999716 ) ) ;
#2378=ORIENTED_EDGE ( 'NONE', *, *, #3700, .T. ) ;
#2379=LINE ( 'NONE', #1057, #5169 ) ;
#2383=VERTEX_POINT ( 'NONE', #5805 ) ;
#2384=ORIENTED_EDGE ( 'NONE', *, *, #3920, .F. ) ;
#2388=CARTESIAN_POINT ( 'NONE',  ( -10.00000000000000000, 28.28427124746189136, -139.9999999999999716 ) ) ;
#2395=DIRECTION ( 'NONE',  ( -1.000000000000000000, 0.000000000000000000, 0.000000000000000000 ) ) ;
#2398=CARTESIAN_POINT ( 'NONE',  ( -5.554394503829287011, 27.95350964898380752, -79.99999999999995737 ) ) ;
#2407=DIRECTION ( 'NONE',  ( -1.000000000000000000, 0.000000000000000000, 0.000000000000000000 ) ) ;
#2411=DIRECTION ( 'NONE',  ( 0.9412010056177179118, 0.3378471059875997051, 1.703375277368107492E-17 ) ) ;
#2412=EDGE_CURVE ( 'NONE', #256, #5216, #4637, .T. ) ;
#2417=CIRCLE ( 'NONE', #636, 29.99999999999999289 ) ;
#2440=VECTOR ( 'NONE', #866, 1000.000000000000000 ) ;
#2448=DIRECTION ( 'NONE',  ( -2.485795968188197231E-17, 1.883273162252411239E-17, 1.000000000000000000 ) ) ;
#2459=EDGE_CURVE ( 'NONE', #6736, #4191, #44, .T. ) ;
#2462=AXIS2_PLACEMENT_3D ( 'NONE', #3274, #6975, #5076 ) ;
#2465=EDGE_LOOP ( 'NONE', ( #2760, #4362, #6266, #2907, #22, #2204, #3465, #6818 ) ) ;
#2469=MECHANICAL_DESIGN_GEOMETRIC_PRESENTATION_REPRESENTATION('',(#180),#5983);
#2476=DIRECTION ( 'NONE',  ( -0.000000000000000000, 0.000000000000000000, -1.000000000000000000 ) ) ;
#2488=VECTOR ( 'NONE', #7113, 1000.000000000000000 ) ;
#2492=ORIENTED_EDGE ( 'NONE', *, *, #558, .F. ) ;
#2497=VECTOR ( 'NONE', #4086, 1000.000000000000000 ) ;
#2504=LINE ( 'NONE', #518, #4314 ) ;
#2506=VECTOR ( 'NONE', #1545, 1000.000000000000000 ) ;
#2519=ADVANCED_FACE ( 'NONE', ( #6083 ), #597, .T. ) ;
#2522=CARTESIAN_POINT ( 'NONE',  ( -35.00000000000000711, 0.000000000000000000, -50.00000000000000000 ) ) ;
#2534=ORIENTED_EDGE ( 'NONE', *, *, #4723, .F. ) ;
#2537=VERTEX_POINT ( 'NONE', #1903 ) ;
#2540=CARTESIAN_POINT ( 'NONE',  ( 35.00000000000000711, 4.286263797015737285E-15, -50.00000000000000000 ) ) ;
#2547=APPLICATION_CONTEXT ( 'automotive_design' ) ;
#2549=DIRECTION ( 'NONE',  ( 0.1303874742813643239, 0.9914631140645255858, 0.000000000000000000 ) ) ;
#2557=ADVANCED_FACE ( 'NONE', ( #2615 ), #3203, .T. ) ;
#2559=VECTOR ( 'NONE', #1879, 1000.000000000000000 ) ;
#2561=SHAPE_REPRESENTATION ( 'Drive Shaft Keyed Hub', ( #7485 ), #7737 ) ;
#2574=EDGE_LOOP ( 'NONE', ( #7203, #5831 ) ) ;
#2597=CARTESIAN_POINT ( 'NONE',  ( 3.911624228440930828, 29.74389342193577690, 10.00000000000000000 ) ) ;
#2602=ORIENTED_EDGE ( 'NONE', *, *, #5971, .F. ) ;
#2606=ORIENTED_EDGE ( 'NONE', *, *, #3920, .T. ) ;
#2612=DIRECTION ( 'NONE',  ( -1.000000000000000000, 0.000000000000000000, 0.000000000000000000 ) ) ;
#2615=FACE_OUTER_BOUND ( 'NONE', #89, .T. ) ;
#2621=DIRECTION ( 'NONE',  ( 0.000000000000000000, 0.000000000000000000, 1.000000000000000000 ) ) ;
#2629=DIRECTION ( 'NONE',  ( 0.000000000000000000, 0.000000000000000000, -1.000000000000000000 ) ) ;
#2632=AXIS2_PLACEMENT_3D ( 'NONE', #3773, #2629, #4395 ) ;
#2637=ADVANCED_FACE ( 'NONE', ( #2064 ), #2689, .F. ) ;
#2640=DIRECTION ( 'NONE',  ( -1.000000000000000000, 0.000000000000000000, 0.000000000000000000 ) ) ;
#2646=VECTOR ( 'NONE', #4284, 1000.000000000000000 ) ;
#2653=ADVANCED_FACE ( 'NONE', ( #7490 ), #7455, .T. ) ;
#2661=DIRECTION ( 'NONE',  ( 3.081487911019577365E-33, -2.775557561562891967E-17, -1.000000000000000000 ) ) ;
#2664=CIRCLE ( 'NONE', #4297, 29.99999999999999289 ) ;
#2668=CARTESIAN_POINT ( 'NONE',  ( -29.99999999999999289, 3.673940397442058389E-15, -79.99999999999995737 ) ) ;
#2678=AXIS2_PLACEMENT_3D ( 'NONE', #7698, #5885, #5135 ) ;
#2679=ORIENTED_EDGE ( 'NONE', *, *, #1727, .T. ) ;
#2680=EDGE_CURVE ( 'NONE', #1325, #5846, #5680, .T. ) ;
#2689=PLANE ( 'NONE',  #981 ) ;
#2700=ORIENTED_EDGE ( 'NONE', *, *, #757, .F. ) ;
#2703=CARTESIAN_POINT ( 'NONE',  ( 10.00000000000000000, 28.28427124746189136, -139.9999999999999716 ) ) ;
#2717=LINE ( 'NONE', #226, #5160 ) ;
#2719=ORIENTED_EDGE ( 'NONE', *, *, #1619, .F. ) ;
#2720=ORIENTED_EDGE ( 'NONE', *, *, #5436, .F. ) ;
#2736=ORIENTED_EDGE ( 'NONE', *, *, #5088, .T. ) ;
#2739=CIRCLE ( 'NONE', #7520, 28.50000000000000711 ) ;
#2743=CARTESIAN_POINT ( 'NONE',  ( 0.000000000000000000, 0.000000000000000000, -60.00000000000000711 ) ) ;
#2760=ORIENTED_EDGE ( 'NONE', *, *, #5823, .T. ) ;
#2768=EDGE_LOOP ( 'NONE', ( #7339, #5182, #3112, #6048 ) ) ;
#2771=CARTESIAN_POINT ( 'NONE',  ( 0.000000000000000000, 0.000000000000000000, 13.00000000000001066 ) ) ;
#2777=ADVANCED_FACE ( 'NONE', ( #5359 ), #6502, .T. ) ;
#2783=CARTESIAN_POINT ( 'NONE',  ( 10.00000000000000000, 33.54101966249685773, -50.00000000000000000 ) ) ;
#2788=CIRCLE ( 'NONE', #883, 28.50000000000000711 ) ;
#2793=ORIENTED_EDGE ( 'NONE', *, *, #1486, .T. ) ;
#2801=ORIENTED_EDGE ( 'NONE', *, *, #1522, .T. ) ;
#2810=DIRECTION ( 'NONE',  ( -0.000000000000000000, -0.000000000000000000, 1.000000000000000000 ) ) ;
#2811=DIRECTION ( 'NONE',  ( 0.000000000000000000, 0.000000000000000000, -1.000000000000000000 ) ) ;
#2820=PLANE ( 'NONE',  #4265 ) ;
#2828=ORIENTED_EDGE ( 'NONE', *, *, #878, .F. ) ;
#2829=ADVANCED_FACE ( 'NONE', ( #3581 ), #4800, .T. ) ;
#2843=CARTESIAN_POINT ( 'NONE',  ( -1.728922298134113098E-15, 8.513302795252935035E-16, 10.00000000000000000 ) ) ;
#2847=EDGE_LOOP ( 'NONE', ( #2720, #6760, #6965, #2679, #6443, #811 ) ) ;
#2871=DIRECTION ( 'NONE',  ( 0.000000000000000000, 0.000000000000000000, 1.000000000000000000 ) ) ;
#2873=CARTESIAN_POINT ( 'NONE',  ( 28.32536770618215982, -3.150165759062971471, 10.00000000000000000 ) ) ;
#2876=ORIENTED_EDGE ( 'NONE', *, *, #2412, .F. ) ;
#2880=DIRECTION ( 'NONE',  ( -5.551115123125782702E-17, 0.000000000000000000, -1.000000000000000000 ) ) ;
#2883=( NAMED_UNIT ( * ) PLANE_ANGLE_UNIT ( ) SI_UNIT ( $, .RADIAN. ) );
#2885=VECTOR ( 'NONE', #1318, 1000.000000000000114 ) ;
#2888=VERTEX_POINT ( 'NONE', #1248 ) ;
#2895=ADVANCED_FACE ( 'NONE', ( #6185, #4361 ), #4993, .T. ) ;
#2907=ORIENTED_EDGE ( 'NONE', *, *, #4259, .F. ) ;
#2932=DIRECTION ( 'NONE',  ( 0.9845265360683707057, 0.1752355551171480841, 0.000000000000000000 ) ) ;
#2943=DIRECTION ( 'NONE',  ( 0.000000000000000000, 0.000000000000000000, 1.000000000000000000 ) ) ;
#2966=AXIS2_PLACEMENT_3D ( 'NONE', #214, #921, #7550 ) ;
#2968=ORIENTED_EDGE ( 'NONE', *, *, #6542, .F. ) ;
#2971=DIRECTION ( 'NONE',  ( -5.551115123125782702E-17, 0.000000000000000000, -1.000000000000000000 ) ) ;
#2972=DIRECTION ( 'NONE',  ( 0.000000000000000000, 0.000000000000000000, 1.000000000000000000 ) ) ;
#2974=ORIENTED_EDGE ( 'NONE', *, *, #5133, .T. ) ;
#2975=EDGE_CURVE ( 'NONE', #1710, #6167, #103, .T. ) ;
#2979=PLANE ( 'NONE',  #5248 ) ;
#2987=ORIENTED_EDGE ( 'NONE', *, *, #5198, .F. ) ;
#2988=VECTOR ( 'NONE', #3643, 1000.000000000000000 ) ;
#2993=VECTOR ( 'NONE', #6884, 1000.000000000000000 ) ;
#3011=VECTOR ( 'NONE', #6575, 1000.000000000000000 ) ;
#3015=ORIENTED_EDGE ( 'NONE', *, *, #2116, .T. ) ;
#3017=ORIENTED_EDGE ( 'NONE', *, *, #4529, .T. ) ;
#3020=PLANE ( 'NONE',  #617 ) ;
#3021=CARTESIAN_POINT ( 'NONE',  ( 3.716043017018883621, 28.25669875083898930, 13.00000000000000178 ) ) ;
#3039=EDGE_LOOP ( 'NONE', ( #118, #3859, #281, #1362 ) ) ;
#3053=DIRECTION ( 'NONE',  ( 3.081487911019577365E-33, -2.775557561562891967E-17, -1.000000000000000000 ) ) ;
#3056=CARTESIAN_POINT ( 'NONE',  ( -28.05900627794857272, -4.994213320838722936, -82.99999999999995737 ) ) ;
#3063=AXIS2_PLACEMENT_3D ( 'NONE', #5416, #3676, #46 ) ;
#3067=PLANE ( 'NONE',  #6521 ) ;
#3098=CYLINDRICAL_SURFACE ( 'NONE', #3437, 29.99999999999999289 ) ;
#3102=CIRCLE ( 'NONE', #823, 28.50000000000000711 ) ;
#3103=ORIENTED_EDGE ( 'NONE', *, *, #6610, .F. ) ;
#3110=DIRECTION ( 'NONE',  ( -1.000000000000000000, 0.000000000000000000, -0.000000000000000000 ) ) ;
#3112=ORIENTED_EDGE ( 'NONE', *, *, #1525, .T. ) ;
#3116=EDGE_LOOP ( 'NONE', ( #3340, #4935, #7333, #635, #613, #2987, #4400, #4921 ) ) ;
#3119=CYLINDRICAL_SURFACE ( 'NONE', #3705, 28.50000000000000711 ) ;
#3123=VERTEX_POINT ( 'NONE', #7057 ) ;
#3127=CARTESIAN_POINT ( 'NONE',  ( -5.846731056662405557, 29.42474699893032053, -82.99999999999995737 ) ) ;
#3137=CARTESIAN_POINT ( 'NONE',  ( -4.665299213380359689, 29.63502966507089909, -82.99999999999995737 ) ) ;
#3142=DIRECTION ( 'NONE',  ( 0.000000000000000000, 0.000000000000000000, 1.000000000000000000 ) ) ;
#3144=VECTOR ( 'NONE', #4044, 1000.000000000000000 ) ;
#3155=ORIENTED_EDGE ( 'NONE', *, *, #2116, .F. ) ;
#3171=CARTESIAN_POINT ( 'NONE',  ( -1.728922298134113098E-15, 8.513302795252935035E-16, 13.00000000000000178 ) ) ;
#3180=EDGE_CURVE ( 'NONE', #6741, #5661, #5794, .T. ) ;
#3192=VERTEX_POINT ( 'NONE', #7257 ) ;
#3203=CYLINDRICAL_SURFACE ( 'NONE', #6281, 29.99999999999999289 ) ;
#3206=ORIENTED_EDGE ( 'NONE', *, *, #707, .T. ) ;
#3211=LINE ( 'NONE', #950, #3883 ) ;
#3218=FACE_OUTER_BOUND ( 'NONE', #2768, .T. ) ;
#3229=ORIENTED_EDGE ( 'NONE', *, *, #5631, .F. ) ;
#3233=FACE_OUTER_BOUND ( 'NONE', #4739, .T. ) ;
#3234=CARTESIAN_POINT ( 'NONE',  ( 0.000000000000000000, 0.000000000000000000, 13.00000000000001066 ) ) ;
#3248=FACE_OUTER_BOUND ( 'NONE', #1409, .T. ) ;
#3253=DIRECTION ( 'NONE',  ( -2.485795968188197231E-17, 1.883273162252411239E-17, 1.000000000000000000 ) ) ;
#3257=LINE ( 'NONE', #6372, #3992 ) ;
#3266=EDGE_CURVE ( 'NONE', #1601, #2088, #7186, .T. ) ;
#3268=AXIS2_PLACEMENT_3D ( 'NONE', #6132, #5797, #6318 ) ;
#3274=CARTESIAN_POINT ( 'NONE',  ( 10.16320117273318679, -26.62629042736811869, -122.9999999999999716 ) ) ;
#3277=VERTEX_POINT ( 'NONE', #3346 ) ;
#3279=FACE_OUTER_BOUND ( 'NONE', #4920, .T. ) ;
#3284=AXIS2_PLACEMENT_3D ( 'NONE', #1106, #2971, #1146 ) ;
#3292=DIRECTION ( 'NONE',  ( 0.000000000000000000, 1.000000000000000000, 0.000000000000000000 ) ) ;
#3293=DIRECTION ( 'NONE',  ( -0.000000000000000000, -0.000000000000000000, -1.000000000000000000 ) ) ;
#3294=CYLINDRICAL_SURFACE ( 'NONE', #4080, 29.99999999999999289 ) ;
#3295=CYLINDRICAL_SURFACE ( 'NONE', #2632, 35.00000000000000711 ) ;
#3300=ORIENTED_EDGE ( 'NONE', *, *, #7014, .F. ) ;
#3303=CYLINDRICAL_SURFACE ( 'NONE', #4976, 35.00000000000000711 ) ;
#3307=DIRECTION ( 'NONE',  ( 3.081487911019577365E-33, -2.775557561562891967E-17, -1.000000000000000000 ) ) ;
#3323=CIRCLE ( 'NONE', #415, 29.99999999999999289 ) ;
#3327=ORIENTED_EDGE ( 'NONE', *, *, #757, .T. ) ;
#3339=ORIENTED_EDGE ( 'NONE', *, *, #7693, .F. ) ;
#3340=ORIENTED_EDGE ( 'NONE', *, *, #6542, .T. ) ;
#3343=DIRECTION ( 'NONE',  ( 1.000000000000000000, 0.000000000000000000, -0.000000000000000000 ) ) ;
#3346=CARTESIAN_POINT ( 'NONE',  ( 2.583028308771596837, 28.38270538120150377, 10.00000000000000000 ) ) ;
#3362=EDGE_CURVE ( 'NONE', #5940, #599, #2717, .T. ) ;
#3367=EDGE_LOOP ( 'NONE', ( #7045, #5697, #2138, #2968 ) ) ;
#3384=DIRECTION ( 'NONE',  ( 0.000000000000000000, 0.000000000000000000, 1.000000000000000000 ) ) ;
#3395=DIRECTION ( 'NONE',  ( -0.000000000000000000, -0.000000000000000000, 1.000000000000000000 ) ) ;
#3397=EDGE_LOOP ( 'NONE', ( #4682, #116, #2736, #7347 ) ) ;
#3405=ORIENTED_EDGE ( 'NONE', *, *, #1443, .F. ) ;
#3413=DIRECTION ( 'NONE',  ( 5.551115123125782702E-17, -0.000000000000000000, 1.000000000000000000 ) ) ;
#3415=ORIENTED_EDGE ( 'NONE', *, *, #3563, .T. ) ;
#3418=DIRECTION ( 'NONE',  ( 0.000000000000000000, 0.000000000000000000, 1.000000000000000000 ) ) ;
#3437=AXIS2_PLACEMENT_3D ( 'NONE', #1232, #3644, #1874 ) ;
#3439=ORIENTED_EDGE ( 'NONE', *, *, #394, .T. ) ;
#3442=CARTESIAN_POINT ( 'NONE',  ( 10.00000000000000000, 41.99999999999999289, -60.00000000000000711 ) ) ;
#3443=VECTOR ( 'NONE', #5516, 1000.000000000000000 ) ;
#3445=FACE_OUTER_BOUND ( 'NONE', #4411, .T. ) ;
#3446=DIRECTION ( 'NONE',  ( -0.09063257223759992043, -0.9958843993404034034, 0.000000000000000000 ) ) ;
#3459=EDGE_CURVE ( 'NONE', #3634, #4724, #1901, .T. ) ;
#3460=FACE_OUTER_BOUND ( 'NONE', #6881, .T. ) ;
#3465=ORIENTED_EDGE ( 'NONE', *, *, #5863, .F. ) ;
#3466=ADVANCED_FACE ( 'NONE', ( #6590 ), #7695, .T. ) ;
#3471=EDGE_CURVE ( 'NONE', #1710, #4364, #2417, .T. ) ;
#3481=CARTESIAN_POINT ( 'NONE',  ( 9.090232026328989079, -27.01143612819398143, -122.9999999999999716 ) ) ;
#3483=ORIENTED_EDGE ( 'NONE', *, *, #1027, .T. ) ;
#3490=CARTESIAN_POINT ( 'NONE',  ( 29.99999999999999289, 0.000000000000000000, 13.00000000000001066 ) ) ;
#3503=EDGE_CURVE ( 'NONE', #6073, #2129, #4538, .T. ) ;
#3513=CARTESIAN_POINT ( 'NONE',  ( 26.82422866010495710, 9.628642520646586433, -122.9999999999999716 ) ) ;
#3516=ORIENTED_EDGE ( 'NONE', *, *, #6493, .F. ) ;
#3538=FACE_OUTER_BOUND ( 'NONE', #5994, .T. ) ;
#3543=ORIENTED_EDGE ( 'NONE', *, *, #4867, .F. ) ;
#3557=CARTESIAN_POINT ( 'NONE',  ( 0.000000000000000000, 0.000000000000000000, -139.9999999999999716 ) ) ;
#3558=DIRECTION ( 'NONE',  ( 0.000000000000000000, -1.000000000000000000, 0.000000000000000000 ) ) ;
#3563=EDGE_CURVE ( 'NONE', #3277, #886, #6054, .T. ) ;
#3567=VECTOR ( 'NONE', #6734, 1000.000000000000000 ) ;
#3574=ORIENTED_EDGE ( 'NONE', *, *, #6844, .T. ) ;
#3575=AXIS2_PLACEMENT_3D ( 'NONE', #778, #7374, #1821 ) ;
#3581=FACE_OUTER_BOUND ( 'NONE', #1892, .T. ) ;
#3599=ADVANCED_FACE ( 'NONE', ( #1224 ), #711, .T. ) ;
#3612=DIRECTION ( 'NONE',  ( 0.000000000000000000, 0.000000000000000000, 1.000000000000000000 ) ) ;
#3615=VERTEX_POINT ( 'NONE', #3127 ) ;
#3619=CIRCLE ( 'NONE', #207, 29.99999999999999289 ) ;
#3620=CARTESIAN_POINT ( 'NONE',  ( 26.82422866010496776, 9.628642520646589986, -122.9999999999999716 ) ) ;
#3621=DIRECTION ( 'NONE',  ( 0.000000000000000000, 0.000000000000000000, -1.000000000000000000 ) ) ;
#3627=VECTOR ( 'NONE', #1206, 1000.000000000000000 ) ;
#3629=ORIENTED_EDGE ( 'NONE', *, *, #558, .T. ) ;
#3634=VERTEX_POINT ( 'NONE', #2540 ) ;
#3643=DIRECTION ( 'NONE',  ( -0.000000000000000000, -0.000000000000000000, -1.000000000000000000 ) ) ;
#3644=DIRECTION ( 'NONE',  ( 0.000000000000000000, 0.000000000000000000, 1.000000000000000000 ) ) ;
#3645=DIRECTION ( 'NONE',  ( -1.000000000000000000, 0.000000000000000000, -0.000000000000000000 ) ) ;
#3652=CARTESIAN_POINT ( 'NONE',  ( -35.00000000000000711, 0.000000000000000000, -60.00000000000000711 ) ) ;
#3659=DIRECTION ( 'NONE',  ( 0.000000000000000000, 0.000000000000000000, -1.000000000000000000 ) ) ;
#3666=LINE ( 'NONE', #74, #1519 ) ;
#3676=DIRECTION ( 'NONE',  ( 3.081487911019577365E-33, -2.775557561562891967E-17, -1.000000000000000000 ) ) ;
#3679=FACE_OUTER_BOUND ( 'NONE', #1173, .T. ) ;
#3685=ADVANCED_FACE ( 'NONE', ( #2142 ), #6390, .T. ) ;
#3691=PLANE ( 'NONE',  #6271 ) ;
#3700=EDGE_CURVE ( 'NONE', #1573, #5335, #1008, .T. ) ;
#3701=VERTEX_POINT ( 'NONE', #939 ) ;
#3705=AXIS2_PLACEMENT_3D ( 'NONE', #1368, #4332, #113 ) ;
#3711=CIRCLE ( 'NONE', #2078, 29.99999999999999289 ) ;
#3731=CARTESIAN_POINT ( 'NONE',  ( 10.16320117273318679, -26.62629042736811869, -122.9999999999999716 ) ) ;
#3734=CIRCLE ( 'NONE', #1465, 29.99999999999999289 ) ;
#3735=CARTESIAN_POINT ( 'NONE',  ( 3.716043017018883621, 28.25669875083898930, 13.00000000000000178 ) ) ;
#3739=ORIENTED_EDGE ( 'NONE', *, *, #5436, .T. ) ;
#3742=ORIENTED_EDGE ( 'NONE', *, *, #6939, .F. ) ;
#3745=EDGE_CURVE ( 'NONE', #599, #6897, #2284, .T. ) ;
#3758=DIRECTION ( 'NONE',  ( 0.000000000000000000, 0.000000000000000000, 1.000000000000000000 ) ) ;
#3761=EDGE_LOOP ( 'NONE', ( #1393, #7371, #3300, #973 ) ) ;
#3765=DIRECTION ( 'NONE',  ( -0.09063257223759993431, -0.9958843993404034034, 0.000000000000000000 ) ) ;
#3771=CARTESIAN_POINT ( 'NONE',  ( 2.583028308771596837, 28.38270538120150377, 13.00000000000000178 ) ) ;
#3773=CARTESIAN_POINT ( 'NONE',  ( 0.000000000000000000, 0.000000000000000000, -50.00000000000000000 ) ) ;
#3774=CARTESIAN_POINT ( 'NONE',  ( 29.99999999999999289, 0.000000000000000000, -139.9999999999999716 ) ) ;
#3775=PRODUCT_CONTEXT ( 'NONE', #7169, 'mechanical' ) ;
#3782=CARTESIAN_POINT ( 'NONE',  ( -10.00000000000000000, 33.54101966249685773, -50.00000000000000000 ) ) ;
#3789=ORIENTED_EDGE ( 'NONE', *, *, #573, .F. ) ;
#3797=CARTESIAN_POINT ( 'NONE',  ( -26.82422866010495710, -9.628642520646591763, -119.9999999999999716 ) ) ;
#3800=ADVANCED_FACE ( 'NONE', ( #3279 ), #6983, .T. ) ;
#3804=CARTESIAN_POINT ( 'NONE',  ( 29.99999999999999289, 0.000000000000000000, -50.00000000000000000 ) ) ;
#3806=ORIENTED_EDGE ( 'NONE', *, *, #4529, .F. ) ;
#3822=DIRECTION ( 'NONE',  ( -1.000000000000000000, 8.881784197001252323E-16, 0.000000000000000000 ) ) ;
#3832=STYLED_ITEM('',(#7830),#5676);
#3837=EDGE_CURVE ( 'NONE', #4532, #3942, #2379, .T. ) ;
#3844=CIRCLE ( 'NONE', #6238, 29.99999999999999289 ) ;
#3845=ORIENTED_EDGE ( 'NONE', *, *, #4042, .F. ) ;
#3848=PLANE ( 'NONE',  #6896 ) ;
#3859=ORIENTED_EDGE ( 'NONE', *, *, #3362, .T. ) ;
#3872=DIRECTION ( 'NONE',  ( 0.000000000000000000, 0.000000000000000000, -1.000000000000000000 ) ) ;
#3874=CIRCLE ( 'NONE', #6713, 28.50000000000000711 ) ;
#3877=CARTESIAN_POINT ( 'NONE',  ( 5.777789833161707559E-31, -4.119912841284263785E-15, -119.9999999999999716 ) ) ;
#3881=VERTEX_POINT ( 'NONE', #5279 ) ;
#3883=VECTOR ( 'NONE', #2621, 1000.000000000000000 ) ;
#3888=DIRECTION ( 'NONE',  ( -1.000000000000000000, 0.000000000000000000, 0.000000000000000000 ) ) ;
#3900=CARTESIAN_POINT ( 'NONE',  ( 5.870234470492294880E-31, -4.203179568131150526E-15, -122.9999999999999716 ) ) ;
#3907=EDGE_CURVE ( 'NONE', #5665, #1972, #6061, .T. ) ;
#3915=CARTESIAN_POINT ( 'NONE',  ( 10.69810649761387822, -28.02767413407169528, -119.9999999999999716 ) ) ;
#3919=CARTESIAN_POINT ( 'NONE',  ( 10.00000000000000000, 28.28427124746189136, -50.00000000000000000 ) ) ;
#3920=EDGE_CURVE ( 'NONE', #952, #387, #7138, .T. ) ;
#3925=ORIENTED_EDGE ( 'NONE', *, *, #7644, .T. ) ;
#3927=EDGE_CURVE ( 'NONE', #6002, #7492, #2788, .T. ) ;
#3941=ORIENTED_EDGE ( 'NONE', *, *, #1377, .F. ) ;
#3942=VERTEX_POINT ( 'NONE', #5514 ) ;
#3947=DIRECTION ( 'NONE',  ( 1.000000000000000000, 0.000000000000000000, 0.000000000000000000 ) ) ;
#3961=DIRECTION ( 'NONE',  ( -0.000000000000000000, -0.000000000000000000, 1.000000000000000000 ) ) ;
#3964=CARTESIAN_POINT ( 'NONE',  ( 0.000000000000000000, 0.000000000000000000, -139.9999999999999716 ) ) ;
#3968=ORIENTED_EDGE ( 'NONE', *, *, #4183, .T. ) ;
#3970=CYLINDRICAL_SURFACE ( 'NONE', #5902, 29.99999999999999289 ) ;
#3975=EDGE_LOOP ( 'NONE', ( #6707, #3483, #2366, #3516 ) ) ;
#3978=EDGE_CURVE ( 'NONE', #2537, #578, #3666, .T. ) ;
#3986=AXIS2_PLACEMENT_3D ( 'NONE', #5802, #6516, #1105 ) ;
#3992=VECTOR ( 'NONE', #249, 1000.000000000000114 ) ;
#4019=LINE ( 'NONE', #4096, #792 ) ;
#4021=CARTESIAN_POINT ( 'NONE',  ( -10.00000000000000000, 0.000000000000000000, 10.00000000000000000 ) ) ;
#4035=CARTESIAN_POINT ( 'NONE',  ( -35.00000000000000711, 0.000000000000000000, -50.00000000000000000 ) ) ;
#4042=EDGE_CURVE ( 'NONE', #886, #5665, #4420, .T. ) ;
#4044=DIRECTION ( 'NONE',  ( -0.000000000000000000, -0.000000000000000000, -1.000000000000000000 ) ) ;
#4056=ORIENTED_EDGE ( 'NONE', *, *, #3471, .F. ) ;
#4059=PRODUCT_DEFINITION_CONTEXT ( 'detailed design', #2547, 'design' ) ;
#4069=AXIS2_PLACEMENT_3D ( 'NONE', #7351, #3395, #385 ) ;
#4077=CARTESIAN_POINT ( 'NONE',  ( -6.873268260756527152E-15, 0.000000000000000000, -79.99999999999995737 ) ) ;
#4080=AXIS2_PLACEMENT_3D ( 'NONE', #4588, #442, #398 ) ;
#4085=LINE ( 'NONE', #6422, #859 ) ;
#4086=DIRECTION ( 'NONE',  ( 0.000000000000000000, 0.000000000000000000, 1.000000000000000000 ) ) ;
#4088=PLANE ( 'NONE',  #6354 ) ;
#4092=ORIENTED_EDGE ( 'NONE', *, *, #6844, .F. ) ;
#4096=CARTESIAN_POINT ( 'NONE',  ( -4.432034252711344102, 28.15327818181735964, -79.99999999999995737 ) ) ;
#4098=ORIENTED_EDGE ( 'NONE', *, *, #6595, .T. ) ;
#4102=CIRCLE ( 'NONE', #452, 29.99999999999999289 ) ;
#4103=DIRECTION ( 'NONE',  ( 5.551115123125782702E-17, 0.000000000000000000, 1.000000000000000000 ) ) ;
#4112=LINE ( 'NONE', #7118, #5410 ) ;
#4121=PLANE ( 'NONE',  #1654 ) ;
#4130=ORIENTED_EDGE ( 'NONE', *, *, #1738, .T. ) ;
#4141=VECTOR ( 'NONE', #3961, 1000.000000000000000 ) ;
#4143=DIRECTION ( 'NONE',  ( 0.000000000000000000, 0.000000000000000000, -1.000000000000000000 ) ) ;
#4145=DIRECTION ( 'NONE',  ( 0.000000000000000000, 0.000000000000000000, -1.000000000000000000 ) ) ;
#4160=VERTEX_POINT ( 'NONE', #3782 ) ;
#4172=ORIENTED_EDGE ( 'NONE', *, *, #6211, .T. ) ;
#4180=ORIENTED_EDGE ( 'NONE', *, *, #1691, .F. ) ;
#4181=ORIENTED_EDGE ( 'NONE', *, *, #3907, .T. ) ;
#4183=EDGE_CURVE ( 'NONE', #5921, #6833, #2664, .T. ) ;
#4191=VERTEX_POINT ( 'NONE', #299 ) ;
#4212=CIRCLE ( 'NONE', #5090, 29.99999999999999289 ) ;
#4216=CARTESIAN_POINT ( 'NONE',  ( 5.870234470492294880E-31, -4.203179568131150526E-15, -122.9999999999999716 ) ) ;
#4224=CARTESIAN_POINT ( 'NONE',  ( 0.000000000000000000, 0.000000000000000000, -139.9999999999999716 ) ) ;
#4225=CARTESIAN_POINT ( 'NONE',  ( 0.000000000000000000, 0.000000000000000000, -139.9999999999999716 ) ) ;
#4227=ORIENTED_EDGE ( 'NONE', *, *, #3700, .F. ) ;
#4231=CARTESIAN_POINT ( 'NONE',  ( -5.846731056662409998, 29.42474699893032763, -139.9999999999999716 ) ) ;
#4243=FACE_OUTER_BOUND ( 'NONE', #4304, .T. ) ;
#4249=VECTOR ( 'NONE', #4832, 1000.000000000000000 ) ;
#4251=VERTEX_POINT ( 'NONE', #6308 ) ;
#4254=AXIS2_PLACEMENT_3D ( 'NONE', #2361, #4747, #7157 ) ;
#4258=AXIS2_PLACEMENT_3D ( 'NONE', #4225, #2972, #6637 ) ;
#4259=EDGE_CURVE ( 'NONE', #3942, #6304, #4525, .T. ) ;
#4260=CARTESIAN_POINT ( 'NONE',  ( -1.728922298134113098E-15, 8.513302795252935035E-16, 10.00000000000000000 ) ) ;
#4261=AXIS2_PLACEMENT_3D ( 'NONE', #4988, #1357, #5657 ) ;
#4265=AXIS2_PLACEMENT_3D ( 'NONE', #1076, #443, #5142 ) ;
#4266=EDGE_LOOP ( 'NONE', ( #1928, #6544, #4181, #4882 ) ) ;
#4284=DIRECTION ( 'NONE',  ( 0.000000000000000000, 0.000000000000000000, 1.000000000000000000 ) ) ;
#4286=CARTESIAN_POINT ( 'NONE',  ( 2.583028308771596837, 28.38270538120150377, 13.00000000000000178 ) ) ;
#4297=AXIS2_PLACEMENT_3D ( 'NONE', #3234, #259, #3822 ) ;
#4300=PLANE ( 'NONE',  #1061 ) ;
#4304=EDGE_LOOP ( 'NONE', ( #4130, #2326, #6379, #2793, #3206, #7261, #4672, #4227 ) ) ;
#4306=CARTESIAN_POINT ( 'NONE',  ( 0.000000000000000000, 0.000000000000000000, -82.99999999999995737 ) ) ;
#4314=VECTOR ( 'NONE', #5968, 1000.000000000000000 ) ;
#4318=CARTESIAN_POINT ( 'NONE',  ( 3.716043017018883621, 28.25669875083898930, 10.00000000000000000 ) ) ;
#4320=SHAPE_DEFINITION_REPRESENTATION ( #1387, #2561 ) ;
#4330=DIRECTION ( 'NONE',  ( 0.000000000000000000, 0.000000000000000000, 1.000000000000000000 ) ) ;
#4332=DIRECTION ( 'NONE',  ( -3.081487911019577365E-33, 2.775557561562891967E-17, 1.000000000000000000 ) ) ;
#4337=ORIENTED_EDGE ( 'NONE', *, *, #2120, .T. ) ;
#4342=DIRECTION ( 'NONE',  ( 0.9938725510941108787, -0.1105321318969463978, 0.000000000000000000 ) ) ;
#4345=EDGE_LOOP ( 'NONE', ( #4092, #1791, #15, #3415 ) ) ;
#4347=CARTESIAN_POINT ( 'NONE',  ( 10.00000000000000000, 0.000000000000000000, -60.00000000000000711 ) ) ;
#4350=CARTESIAN_POINT ( 'NONE',  ( 3.911624228440929940, 29.74389342193576979, -139.9999999999999716 ) ) ;
#4357=FACE_OUTER_BOUND ( 'NONE', #200, .T. ) ;
#4360=DIRECTION ( 'NONE',  ( 0.000000000000000000, 0.000000000000000000, -1.000000000000000000 ) ) ;
#4361=FACE_BOUND ( 'NONE', #7193, .T. ) ;
#4362=ORIENTED_EDGE ( 'NONE', *, *, #6602, .T. ) ;
#4363=EDGE_CURVE ( 'NONE', #6304, #4648, #2171, .T. ) ;
#4364=VERTEX_POINT ( 'NONE', #7593 ) ;
#4366=ORIENTED_EDGE ( 'NONE', *, *, #2209, .F. ) ;
#4370=CARTESIAN_POINT ( 'NONE',  ( 10.00000000000000000, 0.000000000000000000, -60.00000000000000711 ) ) ;
#4374=ADVANCED_FACE ( 'NONE', ( #3460 ), #3970, .T. ) ;
#4375=ORIENTED_EDGE ( 'NONE', *, *, #3927, .F. ) ;
#4379=EDGE_CURVE ( 'NONE', #1483, #7447, #4085, .T. ) ;
#4388=CARTESIAN_POINT ( 'NONE',  ( -10.00000000000000000, 41.99999999999999289, 10.00000000000000000 ) ) ;
#4395=DIRECTION ( 'NONE',  ( -1.000000000000000000, 0.000000000000000000, 0.000000000000000000 ) ) ;
#4400=ORIENTED_EDGE ( 'NONE', *, *, #5088, .F. ) ;
#4411=EDGE_LOOP ( 'NONE', ( #188, #7565, #1521, #4482, #3327, #6749, #1346, #4445, #1287, #4366, #2602, #7679 ) ) ;
#4420=CIRCLE ( 'NONE', #1013, 28.50000000000000711 ) ;
#4421=PLANE ( 'NONE',  #542 ) ;
#4427=DIRECTION ( 'NONE',  ( -1.000000000000000000, 0.000000000000000000, 0.000000000000000000 ) ) ;
#4432=DIRECTION ( 'NONE',  ( 0.9412010056177179118, 0.3378471059875997051, 1.703375277368107492E-17 ) ) ;
#4445=ORIENTED_EDGE ( 'NONE', *, *, #6735, .F. ) ;
#4450=VECTOR ( 'NONE', #1324, 1000.000000000000000 ) ;
#4457=DIRECTION ( 'NONE',  ( -5.551115123125782702E-17, 0.000000000000000000, -1.000000000000000000 ) ) ;
#4460=CARTESIAN_POINT ( 'NONE',  ( -28.32536770618216693, 3.150165759062970583, 13.00000000000000178 ) ) ;
#4461=ORIENTED_EDGE ( 'NONE', *, *, #1727, .F. ) ;
#4462=EDGE_CURVE ( 'NONE', #5216, #194, #7165, .T. ) ;
#4475=DIRECTION ( 'NONE',  ( -0.1555099737793451675, 0.9878343221690302212, -1.110223024625155986E-18 ) ) ;
#4482=ORIENTED_EDGE ( 'NONE', *, *, #672, .F. ) ;
#4503=CARTESIAN_POINT ( 'NONE',  ( 28.05900627794855851, 4.994213320838720271, -79.99999999999995737 ) ) ;
#4525=LINE ( 'NONE', #6934, #6163 ) ;
#4529=EDGE_CURVE ( 'NONE', #1972, #1601, #7166, .T. ) ;
#4532=VERTEX_POINT ( 'NONE', #3731 ) ;
#4538=CIRCLE ( 'NONE', #1511, 29.99999999999999289 ) ;
#4540=PLANE ( 'NONE',  #6355 ) ;
#4548=FACE_OUTER_BOUND ( 'NONE', #1693, .T. ) ;
#4552=EDGE_CURVE ( 'NONE', #5239, #5661, #1205, .T. ) ;
#4560=LINE ( 'NONE', #6968, #4599 ) ;
#4565=FACE_OUTER_BOUND ( 'NONE', #6059, .T. ) ;
#4582=LINE ( 'NONE', #3481, #4687 ) ;
#4584=AXIS2_PLACEMENT_3D ( 'NONE', #3900, #3307, #301 ) ;
#4588=CARTESIAN_POINT ( 'NONE',  ( 0.000000000000000000, 0.000000000000000000, -139.9999999999999716 ) ) ;
#4592=CIRCLE ( 'NONE', #6109, 28.50000000000000355 ) ;
#4599=VECTOR ( 'NONE', #1562, 1000.000000000000000 ) ;
#4606=( NAMED_UNIT ( * ) SI_UNIT ( $, .STERADIAN. ) SOLID_ANGLE_UNIT ( ) );
#4608=EDGE_CURVE ( 'NONE', #587, #6167, #353, .T. ) ;
#4614=( LENGTH_UNIT ( ) NAMED_UNIT ( * ) SI_UNIT ( .MILLI., .METRE. ) );
#4637=CIRCLE ( 'NONE', #6153, 35.00000000000000711 ) ;
#4642=CARTESIAN_POINT ( 'NONE',  ( 28.32536770618216693, -3.150165759062972359, 13.00000000000000178 ) ) ;
#4648=VERTEX_POINT ( 'NONE', #2002 ) ;
#4650=CARTESIAN_POINT ( 'NONE',  ( -5.554394503829287011, 27.95350964898380752, -79.99999999999995737 ) ) ;
#4654=ORIENTED_EDGE ( 'NONE', *, *, #5823, .F. ) ;
#4656=ADVANCED_FACE ( 'NONE', ( #804 ), #3295, .T. ) ;
#4670=DIRECTION ( 'NONE',  ( 0.000000000000000000, 0.000000000000000000, -1.000000000000000000 ) ) ;
#4672=ORIENTED_EDGE ( 'NONE', *, *, #1027, .F. ) ;
#4674=VERTEX_POINT ( 'NONE', #5028 ) ;
#4682=ORIENTED_EDGE ( 'NONE', *, *, #6065, .T. ) ;
#4684=DIRECTION ( 'NONE',  ( -3.081487911019577365E-33, 2.775557561562891967E-17, 1.000000000000000000 ) ) ;
#4686=SHAPE_REPRESENTATION_RELATIONSHIP ( 'NONE' , 'NONE' ,  #2561, #5011 ) ;
#4687=VECTOR ( 'NONE', #7031, 1000.000000000000000 ) ;
#4692=AXIS2_PLACEMENT_3D ( 'NONE', #3171, #3872, #4342 ) ;
#4702=DIRECTION ( 'NONE',  ( -0.000000000000000000, -0.000000000000000000, 1.000000000000000000 ) ) ;
#4723=EDGE_CURVE ( 'NONE', #47, #7320, #5062, .T. ) ;
#4724=VERTEX_POINT ( 'NONE', #4035 ) ;
#4730=DIRECTION ( 'NONE',  ( 0.000000000000000000, -1.000000000000000000, 0.000000000000000000 ) ) ;
#4734=CARTESIAN_POINT ( 'NONE',  ( -10.00000000000000000, 41.99999999999999289, -60.00000000000000711 ) ) ;
#4737=CARTESIAN_POINT ( 'NONE',  ( 0.000000000000000000, 0.000000000000000000, -60.00000000000000711 ) ) ;
#4739=EDGE_LOOP ( 'NONE', ( #1371, #6429, #5250, #4461 ) ) ;
#4747=DIRECTION ( 'NONE',  ( 5.551115123125782702E-17, -0.000000000000000000, 1.000000000000000000 ) ) ;
#4752=EDGE_CURVE ( 'NONE', #256, #1043, #2277, .T. ) ;
#4760=CARTESIAN_POINT ( 'NONE',  ( -1.728922298134113098E-15, 8.513302795252935035E-16, 13.00000000000000178 ) ) ;
#4765=ADVANCED_FACE ( 'NONE', ( #4548 ), #2820, .F. ) ;
#4779=ORIENTED_EDGE ( 'NONE', *, *, #2680, .F. ) ;
#4785=CARTESIAN_POINT ( 'NONE',  ( 29.99999999999999289, 0.000000000000000000, 10.00000000000000888 ) ) ;
#4790=ORIENTED_EDGE ( 'NONE', *, *, #6735, .T. ) ;
#4800=CYLINDRICAL_SURFACE ( 'NONE', #7543, 28.50000000000000355 ) ;
#4811=ORIENTED_EDGE ( 'NONE', *, *, #3266, .F. ) ;
#4816=CIRCLE ( 'NONE', #1806, 29.99999999999999289 ) ;
#4824=AXIS2_PLACEMENT_3D ( 'NONE', #7385, #6131, #4979 ) ;
#4825=CARTESIAN_POINT ( 'NONE',  ( 0.000000000000000000, 0.000000000000000000, -50.00000000000000000 ) ) ;
#4832=DIRECTION ( 'NONE',  ( 0.000000000000000000, 0.000000000000000000, 1.000000000000000000 ) ) ;
#4845=CARTESIAN_POINT ( 'NONE',  ( -10.00000000000000000, 0.000000000000000000, -60.00000000000000711 ) ) ;
#4855=CARTESIAN_POINT ( 'NONE',  ( 0.000000000000000000, 0.000000000000000000, 10.00000000000000888 ) ) ;
#4858=ADVANCED_FACE ( 'NONE', ( #1635 ), #1553, .F. ) ;
#4861=LINE ( 'NONE', #7349, #928 ) ;
#4865=UNCERTAINTY_MEASURE_WITH_UNIT (LENGTH_MEASURE( 1.000000000000000082E-05 ), #5273, 'distance_accuracy_value', 'NONE');
#4867=EDGE_CURVE ( 'NONE', #3881, #1325, #4112, .T. ) ;
#4868=ORIENTED_EDGE ( 'NONE', *, *, #369, .T. ) ;
#4873=LINE ( 'NONE', #2522, #842 ) ;
#4881=UNCERTAINTY_MEASURE_WITH_UNIT (LENGTH_MEASURE( 1.000000000000000082E-05 ), #5796, 'distance_accuracy_value', 'NONE');
#4882=ORIENTED_EDGE ( 'NONE', *, *, #5769, .F. ) ;
#4889=VECTOR ( 'NONE', #7029, 1000.000000000000114 ) ;
#4909=ADVANCED_FACE ( 'NONE', ( #7238 ), #3020, .F. ) ;
#4920=EDGE_LOOP ( 'NONE', ( #5888, #6043, #6299, #2013 ) ) ;
#4921=ORIENTED_EDGE ( 'NONE', *, *, #369, .F. ) ;
#4926=ORIENTED_EDGE ( 'NONE', *, *, #4259, .T. ) ;
#4935=ORIENTED_EDGE ( 'NONE', *, *, #1003, .T. ) ;
#4940=AXIS2_PLACEMENT_3D ( 'NONE', #6986, #1616, #3947 ) ;
#4949=CARTESIAN_POINT ( 'NONE',  ( -1.728922298134113098E-15, 8.513302795252935035E-16, 13.00000000000000178 ) ) ;
#4953=CIRCLE ( 'NONE', #4824, 29.99999999999999289 ) ;
#4966=AXIS2_PLACEMENT_3D ( 'NONE', #6937, #228, #6269 ) ;
#4967=ORIENTED_EDGE ( 'NONE', *, *, #1871, .F. ) ;
#4976=AXIS2_PLACEMENT_3D ( 'NONE', #5702, #224, #2640 ) ;
#4979=DIRECTION ( 'NONE',  ( -1.000000000000000000, -1.776356839400250465E-15, 0.000000000000000000 ) ) ;
#4986=LINE ( 'NONE', #6289, #6137 ) ;
#4988=CARTESIAN_POINT ( 'NONE',  ( 0.000000000000000000, 0.000000000000000000, -60.00000000000000000 ) ) ;
#4989=CARTESIAN_POINT ( 'NONE',  ( 2.718977167127996086, 29.87653198021210343, 13.00000000000001066 ) ) ;
#4993=PLANE ( 'NONE',  #494 ) ;
#5008=VECTOR ( 'NONE', #6528, 1000.000000000000114 ) ;
#5011=ADVANCED_BREP_SHAPE_REPRESENTATION ( '', ( #5676, #7485 ), #7737 ) ;
#5016=AXIS2_PLACEMENT_3D ( 'NONE', #3557, #1147, #5254 ) ;
#5023=ORIENTED_EDGE ( 'NONE', *, *, #4552, .T. ) ;
#5026=CARTESIAN_POINT ( 'NONE',  ( -5.554394503829287011, 27.95350964898380752, -82.99999999999995737 ) ) ;
#5028=CARTESIAN_POINT ( 'NONE',  ( 30.00000000000000355, 0.000000000000000000, 20.00000000000000000 ) ) ;
#5050=LINE ( 'NONE', #4460, #2440 ) ;
#5062=LINE ( 'NONE', #7470, #911 ) ;
#5066=ORIENTED_EDGE ( 'NONE', *, *, #5863, .T. ) ;
#5076=DIRECTION ( 'NONE',  ( 0.3566035499204626702, -0.9342558044690565389, 2.649161120199466423E-17 ) ) ;
#5081=DIRECTION ( 'NONE',  ( 0.000000000000000000, 0.000000000000000000, 1.000000000000000000 ) ) ;
#5088=EDGE_CURVE ( 'NONE', #7447, #2140, #6919, .T. ) ;
#5090=AXIS2_PLACEMENT_3D ( 'NONE', #5588, #1481, #5108 ) ;
#5108=DIRECTION ( 'NONE',  ( 0.000000000000000000, -1.000000000000000000, 0.000000000000000000 ) ) ;
#5110=AXIS2_PLACEMENT_3D ( 'NONE', #284, #7503, #841 ) ;
#5116=DIRECTION ( 'NONE',  ( -5.551115123125782702E-17, 0.000000000000000000, -1.000000000000000000 ) ) ;
#5117=CARTESIAN_POINT ( 'NONE',  ( -10.00000000000000000, 33.54101966249685773, -60.00000000000000711 ) ) ;
#5129=CARTESIAN_POINT ( 'NONE',  ( 0.000000000000000000, 0.000000000000000000, -79.99999999999995737 ) ) ;
#5133=EDGE_CURVE ( 'NONE', #2129, #7603, #5463, .T. ) ;
#5135=DIRECTION ( 'NONE',  ( 1.000000000000000000, 0.000000000000000000, 0.000000000000000000 ) ) ;
#5142=DIRECTION ( 'NONE',  ( -0.000000000000000000, 0.000000000000000000, -1.000000000000000000 ) ) ;
#5159=ORIENTED_EDGE ( 'NONE', *, *, #2368, .T. ) ;
#5160=VECTOR ( 'NONE', #5116, 1000.000000000000000 ) ;
#5169=VECTOR ( 'NONE', #4684, 1000.000000000000000 ) ;
#5176=DIRECTION ( 'NONE',  ( 0.000000000000000000, 0.000000000000000000, 1.000000000000000000 ) ) ;
#5181=FACE_OUTER_BOUND ( 'NONE', #4345, .T. ) ;
#5182=ORIENTED_EDGE ( 'NONE', *, *, #3459, .T. ) ;
#5195=AXIS2_PLACEMENT_3D ( 'NONE', #4855, #1794, #6599 ) ;
#5198=EDGE_CURVE ( 'NONE', #2140, #4648, #3323, .T. ) ;
#5212=( GEOMETRIC_REPRESENTATION_CONTEXT ( 3 ) GLOBAL_UNCERTAINTY_ASSIGNED_CONTEXT ( ( #4865 ) ) GLOBAL_UNIT_ASSIGNED_CONTEXT ( ( #5273, #6425, #4606 ) ) REPRESENTATION_CONTEXT ( 'NONE', 'WORKASPACE' ) );
#5213=CIRCLE ( 'NONE', #7105, 35.00000000000000711 ) ;
#5216=VERTEX_POINT ( 'NONE', #6552 ) ;
#5221=CARTESIAN_POINT ( 'NONE',  ( 10.00000000000000000, 0.000000000000000000, 10.00000000000000000 ) ) ;
#5226=CYLINDRICAL_SURFACE ( 'NONE', #1315, 28.50000000000000711 ) ;
#5237=EDGE_CURVE ( 'NONE', #5972, #7642, #4019, .T. ) ;
#5239=VERTEX_POINT ( 'NONE', #3513 ) ;
#5241=ORIENTED_EDGE ( 'NONE', *, *, #6979, .T. ) ;
#5248=AXIS2_PLACEMENT_3D ( 'NONE', #4347, #6052, #2476 ) ;
#5250=ORIENTED_EDGE ( 'NONE', *, *, #6589, .F. ) ;
#5254=DIRECTION ( 'NONE',  ( 1.000000000000000000, 0.000000000000000000, 0.000000000000000000 ) ) ;
#5273=( LENGTH_UNIT ( ) NAMED_UNIT ( * ) SI_UNIT ( .MILLI., .METRE. ) );
#5277=ORIENTED_EDGE ( 'NONE', *, *, #3503, .T. ) ;
#5279=CARTESIAN_POINT ( 'NONE',  ( -10.00000000000000000, 41.99999999999999289, -60.00000000000000711 ) ) ;
#5290=CARTESIAN_POINT ( 'NONE',  ( 0.000000000000000000, 0.000000000000000000, -50.00000000000000000 ) ) ;
#5291=DIRECTION ( 'NONE',  ( 5.551115123125782702E-17, 0.000000000000000000, 1.000000000000000000 ) ) ;
#5292=AXIS2_PLACEMENT_3D ( 'NONE', #6865, #6943, #1413 ) ;
#5293=CARTESIAN_POINT ( 'NONE',  ( -5.554394503829287011, 27.95350964898380752, -82.99999999999995737 ) ) ;
#5294=ORIENTED_EDGE ( 'NONE', *, *, #2368, .F. ) ;
#5314=CARTESIAN_POINT ( 'NONE',  ( 5.870234470492294880E-31, -4.203179568131150526E-15, -122.9999999999999716 ) ) ;
#5328=DIRECTION ( 'NONE',  ( 5.551115123125782702E-17, 0.000000000000000000, 1.000000000000000000 ) ) ;
#5330=ADVANCED_FACE ( 'NONE', ( #1658 ), #1332, .T. ) ;
#5335=VERTEX_POINT ( 'NONE', #1258 ) ;
#5342=CARTESIAN_POINT ( 'NONE',  ( -29.99999999999999289, 3.673940397442058389E-15, -139.9999999999999716 ) ) ;
#5359=FACE_OUTER_BOUND ( 'NONE', #3116, .T. ) ;
#5370=EDGE_LOOP ( 'NONE', ( #972, #5799, #4790, #4180 ) ) ;
#5371=CARTESIAN_POINT ( 'NONE',  ( 10.00000000000000000, 33.54101966249685773, -50.00000000000000000 ) ) ;
#5375=LINE ( 'NONE', #6084, #6207 ) ;
#5376=ORIENTED_EDGE ( 'NONE', *, *, #3180, .T. ) ;
#5379=EDGE_CURVE ( 'NONE', #387, #599, #6974, .T. ) ;
#5394=EDGE_CURVE ( 'NONE', #5921, #4674, #667, .T. ) ;
#5405=AXIS2_PLACEMENT_3D ( 'NONE', #865, #4457, #6868 ) ;
#5410=VECTOR ( 'NONE', #1716, 1000.000000000000000 ) ;
#5416=CARTESIAN_POINT ( 'NONE',  ( 0.000000000000000000, 0.000000000000000000, -119.9999999999999716 ) ) ;
#5424=CARTESIAN_POINT ( 'NONE',  ( 2.718977167127998307, 29.87653198021212475, 10.00000000000000000 ) ) ;
#5425=LINE ( 'NONE', #1767, #2559 ) ;
#5427=EDGE_CURVE ( 'NONE', #5633, #3881, #1217, .T. ) ;
#5433=LINE ( 'NONE', #3735, #303 ) ;
#5436=EDGE_CURVE ( 'NONE', #256, #1325, #7259, .T. ) ;
#5442=CARTESIAN_POINT ( 'NONE',  ( 29.99999999999999289, 0.000000000000000000, -139.9999999999999716 ) ) ;
#5443=ADVANCED_FACE ( 'NONE', ( #5479 ), #3119, .T. ) ;
#5450=DIRECTION ( 'NONE',  ( -0.000000000000000000, -0.000000000000000000, 1.000000000000000000 ) ) ;
#5453=ORIENTED_EDGE ( 'NONE', *, *, #7454, .T. ) ;
#5463=CIRCLE ( 'NONE', #4069, 29.99999999999999289 ) ;
#5466=DIRECTION ( 'NONE',  ( -0.9878343221690302212, -0.1555099737793451398, 5.550004789056644515E-17 ) ) ;
#5479=FACE_OUTER_BOUND ( 'NONE', #5567, .T. ) ;
#5481=EDGE_CURVE ( 'NONE', #4724, #4160, #6473, .T. ) ;
#5497=CARTESIAN_POINT ( 'NONE',  ( -29.99999999999999289, 3.673940397442058389E-15, -60.00000000000000000 ) ) ;
#5502=CARTESIAN_POINT ( 'NONE',  ( 0.000000000000000000, 0.000000000000000000, -60.00000000000000711 ) ) ;
#5510=AXIS2_PLACEMENT_3D ( 'NONE', #287, #845, #368 ) ;
#5512=UNCERTAINTY_MEASURE_WITH_UNIT (LENGTH_MEASURE( 1.000000000000000082E-05 ), #4614, 'distance_accuracy_value', 'NONE');
#5513=ORIENTED_EDGE ( 'NONE', *, *, #3266, .T. ) ;
#5514=CARTESIAN_POINT ( 'NONE',  ( 10.16320117273318679, -26.62629042736811869, -119.9999999999999716 ) ) ;
#5516=DIRECTION ( 'NONE',  ( 0.000000000000000000, 0.000000000000000000, 1.000000000000000000 ) ) ;
#5520=AXIS2_PLACEMENT_3D ( 'NONE', #6839, #6285, #6916 ) ;
#5526=FACE_OUTER_BOUND ( 'NONE', #7476, .T. ) ;
#5531=DIRECTION ( 'NONE',  ( 5.551115123125782702E-17, -0.000000000000000000, 1.000000000000000000 ) ) ;
#5537=ORIENTED_EDGE ( 'NONE', *, *, #4363, .F. ) ;
#5551=ORIENTED_EDGE ( 'NONE', *, *, #672, .T. ) ;
#5557=ORIENTED_EDGE ( 'NONE', *, *, #2357, .F. ) ;
#5563=CARTESIAN_POINT ( 'NONE',  ( 0.000000000000000000, 0.000000000000000000, -139.9999999999999716 ) ) ;
#5567=EDGE_LOOP ( 'NONE', ( #726, #2340, #7242, #5066 ) ) ;
#5583=LINE ( 'NONE', #2703, #6883 ) ;
#5588=CARTESIAN_POINT ( 'NONE',  ( 0.000000000000000000, 0.000000000000000000, -119.9999999999999716 ) ) ;
#5593=ORIENTED_EDGE ( 'NONE', *, *, #3837, .T. ) ;
#5594=CIRCLE ( 'NONE', #4584, 28.50000000000000711 ) ;
#5599=CIRCLE ( 'NONE', #2966, 28.50000000000000711 ) ;
#5617=ADVANCED_FACE ( 'NONE', ( #4565 ), #5706, .F. ) ;
#5629=ORIENTED_EDGE ( 'NONE', *, *, #3837, .F. ) ;
#5631=EDGE_CURVE ( 'NONE', #7368, #5239, #5594, .T. ) ;
#5632=AXIS2_PLACEMENT_3D ( 'NONE', #4734, #6556, #5965 ) ;
#5633=VERTEX_POINT ( 'NONE', #5117 ) ;
#5650=DIRECTION ( 'NONE',  ( -3.081487911019577365E-33, 2.775557561562891967E-17, 1.000000000000000000 ) ) ;
#5657=DIRECTION ( 'NONE',  ( -1.000000000000000000, 0.000000000000000000, 0.000000000000000000 ) ) ;
#5661=VERTEX_POINT ( 'NONE', #1689 ) ;
#5662=EDGE_LOOP ( 'NONE', ( #6350, #626, #2048, #3017 ) ) ;
#5665=VERTEX_POINT ( 'NONE', #2873 ) ;
#5673=ORIENTED_EDGE ( 'NONE', *, *, #512, .T. ) ;
#5674=ADVANCED_FACE ( 'NONE', ( #7088 ), #4088, .T. ) ;
#5675=ORIENTED_EDGE ( 'NONE', *, *, #897, .T. ) ;
#5676=MANIFOLD_SOLID_BREP ( 'Cavity1', #1446 ) ;
#5680=LINE ( 'NONE', #270, #6159 ) ;
#5682=CYLINDRICAL_SURFACE ( 'NONE', #4692, 28.50000000000000711 ) ;
#5683=ORIENTED_EDGE ( 'NONE', *, *, #7357, .T. ) ;
#5692=LINE ( 'NONE', #2276, #681 ) ;
#5697=ORIENTED_EDGE ( 'NONE', *, *, #6639, .T. ) ;
#5702=CARTESIAN_POINT ( 'NONE',  ( 0.000000000000000000, 0.000000000000000000, -50.00000000000000000 ) ) ;
#5706=PLANE ( 'NONE',  #2462 ) ;
#5722=CIRCLE ( 'NONE', #2085, 29.99999999999999289 ) ;
#5725=CARTESIAN_POINT ( 'NONE',  ( 29.99999999999999289, 2.565854121688507820E-48, -122.9999999999999716 ) ) ;
#5745=CIRCLE ( 'NONE', #1591, 28.50000000000000355 ) ;
#5750=ORIENTED_EDGE ( 'NONE', *, *, #7701, .F. ) ;
#5753=ORIENTED_EDGE ( 'NONE', *, *, #3745, .F. ) ;
#5763=DIRECTION ( 'NONE',  ( 1.000000000000000000, 0.000000000000000000, -0.000000000000000000 ) ) ;
#5769=EDGE_CURVE ( 'NONE', #2049, #1972, #5433, .T. ) ;
#5786=DIRECTION ( 'NONE',  ( 1.000000000000000000, 0.000000000000000000, 0.000000000000000000 ) ) ;
#5794=CIRCLE ( 'NONE', #2030, 28.50000000000000711 ) ;
#5796=( LENGTH_UNIT ( ) NAMED_UNIT ( * ) SI_UNIT ( .MILLI., .METRE. ) );
#5797=DIRECTION ( 'NONE',  ( 3.081487911019577365E-33, -2.775557561562891967E-17, -1.000000000000000000 ) ) ;
#5799=ORIENTED_EDGE ( 'NONE', *, *, #3471, .T. ) ;
#5802=CARTESIAN_POINT ( 'NONE',  ( 5.870234470492294880E-31, -4.203179568131150526E-15, -122.9999999999999716 ) ) ;
#5805=CARTESIAN_POINT ( 'NONE',  ( -10.00000000000000000, 41.99999999999999289, 10.00000000000000000 ) ) ;
#5818=DIRECTION ( 'NONE',  ( 0.9845265360683707057, 0.1752355551171480841, 0.000000000000000000 ) ) ;
#5819=ORIENTED_EDGE ( 'NONE', *, *, #48, .T. ) ;
#5823=EDGE_CURVE ( 'NONE', #578, #1051, #4212, .T. ) ;
#5825=CARTESIAN_POINT ( 'NONE',  ( 0.000000000000000000, 0.000000000000000000, -139.9999999999999716 ) ) ;
#5831=ORIENTED_EDGE ( 'NONE', *, *, #6493, .T. ) ;
#5837=LINE ( 'NONE', #7687, #3567 ) ;
#5844=CARTESIAN_POINT ( 'NONE',  ( -6.873268260756527152E-15, 0.000000000000000000, -79.99999999999995737 ) ) ;
#5846=VERTEX_POINT ( 'NONE', #6296 ) ;
#5863=EDGE_CURVE ( 'NONE', #2201, #6741, #5599, .T. ) ;
#5866=DIRECTION ( 'NONE',  ( 0.000000000000000000, 0.000000000000000000, 1.000000000000000000 ) ) ;
#5867=CARTESIAN_POINT ( 'NONE',  ( 5.870234470492294880E-31, -4.203179568131150526E-15, -122.9999999999999716 ) ) ;
#5869=DIRECTION ( 'NONE',  ( 0.9845265360683708167, 0.1752355551171481118, -5.551115123125782086E-17 ) ) ;
#5871=ADVANCED_FACE ( 'NONE', ( #7509 ), #252, .T. ) ;
#5876=DIRECTION ( 'NONE',  ( 0.9938725510941108787, -0.1105321318969463978, 0.000000000000000000 ) ) ;
#5883=DIRECTION ( 'NONE',  ( -1.000000000000000000, 0.000000000000000000, 0.000000000000000000 ) ) ;
#5885=DIRECTION ( 'NONE',  ( 0.000000000000000000, 0.000000000000000000, 1.000000000000000000 ) ) ;
#5888=ORIENTED_EDGE ( 'NONE', *, *, #7317, .T. ) ;
#5896=ORIENTED_EDGE ( 'NONE', *, *, #3459, .F. ) ;
#5902=AXIS2_PLACEMENT_3D ( 'NONE', #5825, #3384, #5786 ) ;
#5904=LINE ( 'NONE', #6456, #2497 ) ;
#5921=VERTEX_POINT ( 'NONE', #3490 ) ;
#5940=VERTEX_POINT ( 'NONE', #1119 ) ;
#5941=DIRECTION ( 'NONE',  ( 0.9845265360683708167, 0.1752355551171481118, -5.551115123125782086E-17 ) ) ;
#5944=DIRECTION ( 'NONE',  ( 0.9412010056177179118, 0.3378471059875997051, 0.000000000000000000 ) ) ;
#5947=DIRECTION ( 'NONE',  ( -5.551115123125782702E-17, 0.000000000000000000, -1.000000000000000000 ) ) ;
#5963=ADVANCED_FACE ( 'NONE', ( #5181 ), #5226, .T. ) ;
#5964=EDGE_CURVE ( 'NONE', #2183, #5972, #4592, .T. ) ;
#5965=DIRECTION ( 'NONE',  ( 0.000000000000000000, -0.000000000000000000, -1.000000000000000000 ) ) ;
#5968=DIRECTION ( 'NONE',  ( 0.000000000000000000, 0.000000000000000000, 1.000000000000000000 ) ) ;
#5971=EDGE_CURVE ( 'NONE', #6819, #7320, #5722, .T. ) ;
#5972=VERTEX_POINT ( 'NONE', #1039 ) ;
#5977=DIRECTION ( 'NONE',  ( 1.000000000000000000, 0.000000000000000000, 0.000000000000000000 ) ) ;
#5983=( GEOMETRIC_REPRESENTATION_CONTEXT ( 3 ) GLOBAL_UNCERTAINTY_ASSIGNED_CONTEXT ( ( #5512 ) ) GLOBAL_UNIT_ASSIGNED_CONTEXT ( ( #4614, #2883, #2300 ) ) REPRESENTATION_CONTEXT ( 'NONE', 'WORKASPACE' ) );
#5994=EDGE_LOOP ( 'NONE', ( #3229, #6613, #5376, #6388 ) ) ;
#6002=VERTEX_POINT ( 'NONE', #2243 ) ;
#6013=CARTESIAN_POINT ( 'NONE',  ( 9.568665290872615969, -28.43309066125680928, -119.9999999999999716 ) ) ;
#6043=ORIENTED_EDGE ( 'NONE', *, *, #400, .T. ) ;
#6048=ORIENTED_EDGE ( 'NONE', *, *, #4462, .F. ) ;
#6052=DIRECTION ( 'NONE',  ( 1.000000000000000000, 0.000000000000000000, -0.000000000000000000 ) ) ;
#6054=CIRCLE ( 'NONE', #1134, 28.50000000000000711 ) ;
#6059=EDGE_LOOP ( 'NONE', ( #304, #6316, #5593, #4926 ) ) ;
#6061=CIRCLE ( 'NONE', #382, 28.50000000000000711 ) ;
#6065=EDGE_CURVE ( 'NONE', #3701, #1483, #3844, .T. ) ;
#6073=VERTEX_POINT ( 'NONE', #6612 ) ;
#6078=DIRECTION ( 'NONE',  ( 0.9412010056177179118, 0.3378471059875997051, 0.000000000000000000 ) ) ;
#6083=FACE_OUTER_BOUND ( 'NONE', #6593, .T. ) ;
#6084=CARTESIAN_POINT ( 'NONE',  ( 9.090232026328989079, -27.01143612819398143, -119.9999999999999716 ) ) ;
#6090=FACE_OUTER_BOUND ( 'NONE', #3975, .T. ) ;
#6106=ORIENTED_EDGE ( 'NONE', *, *, #6589, .T. ) ;
#6109=AXIS2_PLACEMENT_3D ( 'NONE', #4077, #960, #5818 ) ;
#6131=DIRECTION ( 'NONE',  ( -0.000000000000000000, -0.000000000000000000, 1.000000000000000000 ) ) ;
#6132=CARTESIAN_POINT ( 'NONE',  ( 0.000000000000000000, 0.000000000000000000, -122.9999999999999716 ) ) ;
#6137=VECTOR ( 'NONE', #3292, 1000.000000000000000 ) ;
#6153=AXIS2_PLACEMENT_3D ( 'NONE', #4737, #4145, #6558 ) ;
#6155=ORIENTED_EDGE ( 'NONE', *, *, #1691, .T. ) ;
#6156=EDGE_LOOP ( 'NONE', ( #5551, #6791, #2384, #4967 ) ) ;
#6159=VECTOR ( 'NONE', #2214, 1000.000000000000000 ) ;
#6163=VECTOR ( 'NONE', #929, 1000.000000000000114 ) ;
#6167=VERTEX_POINT ( 'NONE', #5497 ) ;
#6177=CARTESIAN_POINT ( 'NONE',  ( 29.99999999999999289, 2.565854121688507820E-48, -119.9999999999999716 ) ) ;
#6185=FACE_OUTER_BOUND ( 'NONE', #2847, .T. ) ;
#6188=ORIENTED_EDGE ( 'NONE', *, *, #1958, .F. ) ;
#6193=DIRECTION ( 'NONE',  ( -0.000000000000000000, 1.000000000000000000, 0.000000000000000000 ) ) ;
#6206=LINE ( 'NONE', #4388, #2506 ) ;
#6207=VECTOR ( 'NONE', #6209, 1000.000000000000000 ) ;
#6209=DIRECTION ( 'NONE',  ( -0.3189555096957539804, 0.9477696887085605981, -2.581026109104742702E-17 ) ) ;
#6211=EDGE_CURVE ( 'NONE', #5335, #4251, #5425, .T. ) ;
#6214=CARTESIAN_POINT ( 'NONE',  ( -29.99999999999999289, 3.673940397442058389E-15, -119.9999999999999716 ) ) ;
#6222=AXIS2_PLACEMENT_3D ( 'NONE', #4216, #1897, #6078 ) ;
#6230=CARTESIAN_POINT ( 'NONE',  ( 5.777789833161707559E-31, -4.119912841284263785E-15, -119.9999999999999716 ) ) ;
#6238=AXIS2_PLACEMENT_3D ( 'NONE', #3964, #3142, #1915 ) ;
#6245=DIRECTION ( 'NONE',  ( -1.000000000000000000, -8.881784197001252323E-16, 0.000000000000000000 ) ) ;
#6246=FACE_BOUND ( 'NONE', #1938, .T. ) ;
#6251=LINE ( 'NONE', #915, #2993 ) ;
#6255=DIRECTION ( 'NONE',  ( 0.000000000000000000, 0.000000000000000000, -1.000000000000000000 ) ) ;
#6257=AXIS2_PLACEMENT_3D ( 'NONE', #2032, #6874, #6913 ) ;
#6263=ORIENTED_EDGE ( 'NONE', *, *, #5394, .F. ) ;
#6266=ORIENTED_EDGE ( 'NONE', *, *, #6610, .T. ) ;
#6269=DIRECTION ( 'NONE',  ( -1.000000000000000000, 0.000000000000000000, 0.000000000000000000 ) ) ;
#6271=AXIS2_PLACEMENT_3D ( 'NONE', #6775, #5466, #770 ) ;
#6279=DIRECTION ( 'NONE',  ( 0.9477696887085605981, 0.3189555096957539804, 1.755346904044972688E-17 ) ) ;
#6281=AXIS2_PLACEMENT_3D ( 'NONE', #5563, #750, #2253 ) ;
#6285=DIRECTION ( 'NONE',  ( -0.000000000000000000, -0.000000000000000000, 1.000000000000000000 ) ) ;
#6286=DIRECTION ( 'NONE',  ( 0.000000000000000000, 0.000000000000000000, -1.000000000000000000 ) ) ;
#6289=CARTESIAN_POINT ( 'NONE',  ( -10.00000000000000000, 0.000000000000000000, -50.00000000000000000 ) ) ;
#6292=LINE ( 'NONE', #6998, #6981 ) ;
#6296=CARTESIAN_POINT ( 'NONE',  ( 10.00000000000000000, 41.99999999999999289, 10.00000000000000000 ) ) ;
#6299=ORIENTED_EDGE ( 'NONE', *, *, #6595, .F. ) ;
#6304=VERTEX_POINT ( 'NONE', #3915 ) ;
#6308=CARTESIAN_POINT ( 'NONE',  ( -30.00000000000000711, 3.673940397442059967E-15, 20.00000000000000000 ) ) ;
#6309=CARTESIAN_POINT ( 'NONE',  ( 0.000000000000000000, 0.000000000000000000, 10.00000000000000000 ) ) ;
#6316=ORIENTED_EDGE ( 'NONE', *, *, #2264, .F. ) ;
#6318=DIRECTION ( 'NONE',  ( 0.000000000000000000, -1.000000000000000000, 0.000000000000000000 ) ) ;
#6338=CIRCLE ( 'NONE', #4940, 30.00000000000000355 ) ;
#6341=CARTESIAN_POINT ( 'NONE',  ( 0.000000000000000000, 0.000000000000000000, -139.9999999999999716 ) ) ;
#6350=ORIENTED_EDGE ( 'NONE', *, *, #2069, .T. ) ;
#6352=ADVANCED_FACE ( 'NONE', ( #279 ), #2036, .T. ) ;
#6354=AXIS2_PLACEMENT_3D ( 'NONE', #7010, #6501, #5869 ) ;
#6355=AXIS2_PLACEMENT_3D ( 'NONE', #7461, #2071, #5763 ) ;
#6372=CARTESIAN_POINT ( 'NONE',  ( 2.583028308771596837, 28.38270538120150377, 13.00000000000000178 ) ) ;
#6374=DIRECTION ( 'NONE',  ( 0.9938725510941108787, -0.1105321318969463978, 0.000000000000000000 ) ) ;
#6379=ORIENTED_EDGE ( 'NONE', *, *, #3927, .T. ) ;
#6387=AXIS2_PLACEMENT_3D ( 'NONE', #2771, #2810, #2266 ) ;
#6388=ORIENTED_EDGE ( 'NONE', *, *, #4552, .F. ) ;
#6390=PLANE ( 'NONE',  #6435 ) ;
#6391=PRESENTATION_STYLE_ASSIGNMENT (( #7685 ) ) ;
#6392=VECTOR ( 'NONE', #692, 1000.000000000000000 ) ;
#6395=EDGE_CURVE ( 'NONE', #3123, #2201, #1392, .T. ) ;
#6403=CARTESIAN_POINT ( 'NONE',  ( 10.16320117273318679, -26.62629042736811869, -122.9999999999999716 ) ) ;
#6410=CARTESIAN_POINT ( 'NONE',  ( 35.00000000000000711, 4.286263797015737285E-15, -50.00000000000000000 ) ) ;
#6422=CARTESIAN_POINT ( 'NONE',  ( -29.99999999999999289, 3.673940397442058389E-15, -139.9999999999999716 ) ) ;
#6425=( NAMED_UNIT ( * ) PLANE_ANGLE_UNIT ( ) SI_UNIT ( $, .RADIAN. ) );
#6429=ORIENTED_EDGE ( 'NONE', *, *, #5481, .T. ) ;
#6433=DIRECTION ( 'NONE',  ( -0.000000000000000000, 1.000000000000000000, 0.000000000000000000 ) ) ;
#6435=AXIS2_PLACEMENT_3D ( 'NONE', #7526, #1497, #861 ) ;
#6443=ORIENTED_EDGE ( 'NONE', *, *, #5427, .T. ) ;
#6445=DIRECTION ( 'NONE',  ( -0.000000000000000000, 1.000000000000000000, 0.000000000000000000 ) ) ;
#6449=DIRECTION ( 'NONE',  ( -1.000000000000000000, 0.000000000000000000, 0.000000000000000000 ) ) ;
#6456=CARTESIAN_POINT ( 'NONE',  ( -29.99999999999999289, 3.673940397442058389E-15, -139.9999999999999716 ) ) ;
#6459=EDGE_CURVE ( 'NONE', #3615, #387, #1588, .T. ) ;
#6464=DIRECTION ( 'NONE',  ( 0.9938725510941108787, -0.1105321318969463978, 0.000000000000000000 ) ) ;
#6466=( NAMED_UNIT ( * ) SI_UNIT ( $, .STERADIAN. ) SOLID_ANGLE_UNIT ( ) );
#6467=CARTESIAN_POINT ( 'NONE',  ( 0.000000000000000000, 0.000000000000000000, -122.9999999999999716 ) ) ;
#6472=DIRECTION ( 'NONE',  ( -1.000000000000000000, 0.000000000000000000, 0.000000000000000000 ) ) ;
#6473=CIRCLE ( 'NONE', #4966, 35.00000000000000711 ) ;
#6475=FACE_OUTER_BOUND ( 'NONE', #3397, .T. ) ;
#6477=ORIENTED_EDGE ( 'NONE', *, *, #1290, .T. ) ;
#6478=PRODUCT_DEFINITION ( 'UNKNOWN', '', #783, #4059 ) ;
#6484=CARTESIAN_POINT ( 'NONE',  ( 3.716043017018883621, 28.25669875083898930, 13.00000000000000178 ) ) ;
#6493=EDGE_CURVE ( 'NONE', #4251, #4674, #7458, .T. ) ;
#6495=DIRECTION ( 'NONE',  ( 0.9938725510941108787, -0.1105321318969463978, 0.000000000000000000 ) ) ;
#6501=DIRECTION ( 'NONE',  ( -5.635681009894454322E-17, -1.505185443864239327E-19, -1.000000000000000000 ) ) ;
#6502=PLANE ( 'NONE',  #4 ) ;
#6504=EDGE_CURVE ( 'NONE', #1573, #2088, #7107, .T. ) ;
#6506=EDGE_LOOP ( 'NONE', ( #2828, #5023, #4337, #5629 ) ) ;
#6511=CIRCLE ( 'NONE', #3986, 28.50000000000000711 ) ;
#6515=AXIS2_PLACEMENT_3D ( 'NONE', #5867, #1047, #5944 ) ;
#6516=DIRECTION ( 'NONE',  ( 3.081487911019577365E-33, -2.775557561562891967E-17, -1.000000000000000000 ) ) ;
#6517=DIRECTION ( 'NONE',  ( -0.000000000000000000, -0.000000000000000000, 1.000000000000000000 ) ) ;
#6521=AXIS2_PLACEMENT_3D ( 'NONE', #4949, #1964, #1848 ) ;
#6528=DIRECTION ( 'NONE',  ( 0.1948910352220799280, -0.9808248999643441879, -1.110223024625155793E-18 ) ) ;
#6532=VERTEX_POINT ( 'NONE', #1108 ) ;
#6542=EDGE_CURVE ( 'NONE', #2537, #3123, #4582, .T. ) ;
#6544=ORIENTED_EDGE ( 'NONE', *, *, #1443, .T. ) ;
#6552=CARTESIAN_POINT ( 'NONE',  ( 35.00000000000000711, 4.286263797015737285E-15, -60.00000000000000711 ) ) ;
#6556=DIRECTION ( 'NONE',  ( 0.000000000000000000, -1.000000000000000000, 0.000000000000000000 ) ) ;
#6558=DIRECTION ( 'NONE',  ( -1.000000000000000000, 0.000000000000000000, 0.000000000000000000 ) ) ;
#6575=DIRECTION ( 'NONE',  ( -3.081487911019577365E-33, 2.775557561562891967E-17, 1.000000000000000000 ) ) ;
#6581=VECTOR ( 'NONE', #5650, 1000.000000000000000 ) ;
#6582=ORIENTED_EDGE ( 'NONE', *, *, #1140, .T. ) ;
#6589=EDGE_CURVE ( 'NONE', #5633, #4160, #6674, .T. ) ;
#6590=FACE_OUTER_BOUND ( 'NONE', #3039, .T. ) ;
#6593=EDGE_LOOP ( 'NONE', ( #1833, #5277, #2801, #344 ) ) ;
#6595=EDGE_CURVE ( 'NONE', #6736, #6532, #1672, .T. ) ;
#6599=DIRECTION ( 'NONE',  ( -1.000000000000000000, -1.776356839400250465E-15, 0.000000000000000000 ) ) ;
#6602=EDGE_CURVE ( 'NONE', #1051, #1102, #4816, .T. ) ;
#6610=EDGE_CURVE ( 'NONE', #1102, #6304, #1162, .T. ) ;
#6612=CARTESIAN_POINT ( 'NONE',  ( -29.99999999999999289, 3.673940397442058389E-15, -50.00000000000000000 ) ) ;
#6613=ORIENTED_EDGE ( 'NONE', *, *, #6984, .T. ) ;
#6614=VECTOR ( 'NONE', #2943, 1000.000000000000000 ) ;
#6637=DIRECTION ( 'NONE',  ( 1.000000000000000000, 0.000000000000000000, 0.000000000000000000 ) ) ;
#6639=EDGE_CURVE ( 'NONE', #578, #2201, #5375, .T. ) ;
#6670=ORIENTED_EDGE ( 'NONE', *, *, #6979, .F. ) ;
#6672=DIRECTION ( 'NONE',  ( 0.000000000000000000, 0.000000000000000000, 1.000000000000000000 ) ) ;
#6674=LINE ( 'NONE', #7306, #2184 ) ;
#6681=AXIS2_PLACEMENT_3D ( 'NONE', #7653, #4143, #2267 ) ;
#6692=CARTESIAN_POINT ( 'NONE',  ( -10.00000000000000000, 41.99999999999999289, -60.00000000000000711 ) ) ;
#6707=ORIENTED_EDGE ( 'NONE', *, *, #6211, .F. ) ;
#6713=AXIS2_PLACEMENT_3D ( 'NONE', #4760, #2871, #7167 ) ;
#6714=ORIENTED_EDGE ( 'NONE', *, *, #2209, .T. ) ;
#6717=DIRECTION ( 'NONE',  ( 5.551115123125782702E-17, -0.000000000000000000, 1.000000000000000000 ) ) ;
#6718=VECTOR ( 'NONE', #6433, 1000.000000000000000 ) ;
#6734=DIRECTION ( 'NONE',  ( -3.081487911019577365E-33, 2.775557561562891967E-17, 1.000000000000000000 ) ) ;
#6735=EDGE_CURVE ( 'NONE', #4364, #587, #2504, .T. ) ;
#6736=VERTEX_POINT ( 'NONE', #559 ) ;
#6737=ADVANCED_FACE ( 'NONE', ( #5526 ), #5682, .T. ) ;
#6741=VERTEX_POINT ( 'NONE', #3797 ) ;
#6749=ORIENTED_EDGE ( 'NONE', *, *, #2975, .T. ) ;
#6751=EDGE_LOOP ( 'NONE', ( #2378, #4172, #3742, #6263, #3968, #2022, #5513, #2021 ) ) ;
#6757=DIRECTION ( 'NONE',  ( -0.000000000000000000, -0.000000000000000000, -1.000000000000000000 ) ) ;
#6759=CARTESIAN_POINT ( 'NONE',  ( 29.99999999999999289, 0.000000000000000000, -82.99999999999995737 ) ) ;
#6760=ORIENTED_EDGE ( 'NONE', *, *, #2412, .T. ) ;
#6769=CIRCLE ( 'NONE', #6387, 29.99999999999999289 ) ;
#6775=CARTESIAN_POINT ( 'NONE',  ( -4.432034252711344102, 28.15327818181735964, -79.99999999999995737 ) ) ;
#6780=VECTOR ( 'NONE', #3612, 1000.000000000000000 ) ;
#6790=ADVANCED_FACE ( 'NONE', ( #751 ), #4421, .F. ) ;
#6791=ORIENTED_EDGE ( 'NONE', *, *, #6459, .T. ) ;
#6817=AXIS2_PLACEMENT_3D ( 'NONE', #4224, #6672, #1300 ) ;
#6818=ORIENTED_EDGE ( 'NONE', *, *, #6639, .F. ) ;
#6819=VERTEX_POINT ( 'NONE', #6759 ) ;
#6831=DIRECTION ( 'NONE',  ( 0.9808248999643442989, 0.1948910352220800113, -5.550004789056643899E-17 ) ) ;
#6833=VERTEX_POINT ( 'NONE', #1382 ) ;
#6839=CARTESIAN_POINT ( 'NONE',  ( 0.000000000000000000, 0.000000000000000000, 10.00000000000000888 ) ) ;
#6844=EDGE_CURVE ( 'NONE', #6002, #886, #5050, .T. ) ;
#6845=CARTESIAN_POINT ( 'NONE',  ( 5.777789833161707559E-31, -4.119912841284263785E-15, -119.9999999999999716 ) ) ;
#6847=DIRECTION ( 'NONE',  ( 0.000000000000000000, 0.000000000000000000, -1.000000000000000000 ) ) ;
#6864=VERTEX_POINT ( 'NONE', #2303 ) ;
#6865=CARTESIAN_POINT ( 'NONE',  ( -7.039801714450301422E-15, 0.000000000000000000, -82.99999999999995737 ) ) ;
#6868=DIRECTION ( 'NONE',  ( 0.9845265360683707057, 0.1752355551171480841, 0.000000000000000000 ) ) ;
#6874=DIRECTION ( 'NONE',  ( 3.081487911019577365E-33, -2.775557561562891967E-17, -1.000000000000000000 ) ) ;
#6876=AXIS2_PLACEMENT_3D ( 'NONE', #876, #6847, #247 ) ;
#6881=EDGE_LOOP ( 'NONE', ( #7500, #3629, #7530, #7142, #5537, #3103, #3925, #3789, #3941, #4654, #165, #4868 ) ) ;
#6883=VECTOR ( 'NONE', #3293, 1000.000000000000000 ) ;
#6884=DIRECTION ( 'NONE',  ( -5.551115123125782702E-17, 0.000000000000000000, -1.000000000000000000 ) ) ;
#6896=AXIS2_PLACEMENT_3D ( 'NONE', #6845, #3253, #4432 ) ;
#6897=VERTEX_POINT ( 'NONE', #349 ) ;
#6905=ORIENTED_EDGE ( 'NONE', *, *, #4608, .T. ) ;
#6912=CIRCLE ( 'NONE', #480, 28.50000000000000355 ) ;
#6913=DIRECTION ( 'NONE',  ( 0.9412010056177179118, 0.3378471059875997051, 0.000000000000000000 ) ) ;
#6916=DIRECTION ( 'NONE',  ( -1.000000000000000000, 0.000000000000000000, 0.000000000000000000 ) ) ;
#6919=CIRCLE ( 'NONE', #3268, 29.99999999999999289 ) ;
#6934=CARTESIAN_POINT ( 'NONE',  ( 10.16320117273318679, -26.62629042736811869, -119.9999999999999716 ) ) ;
#6937=CARTESIAN_POINT ( 'NONE',  ( 0.000000000000000000, 0.000000000000000000, -50.00000000000000000 ) ) ;
#6938=ORIENTED_EDGE ( 'NONE', *, *, #4042, .T. ) ;
#6939=EDGE_CURVE ( 'NONE', #4674, #4251, #6338, .T. ) ;
#6943=DIRECTION ( 'NONE',  ( 5.551115123125782702E-17, 0.000000000000000000, 1.000000000000000000 ) ) ;
#6953=ORIENTED_EDGE ( 'NONE', *, *, #1871, .T. ) ;
#6965=ORIENTED_EDGE ( 'NONE', *, *, #4462, .T. ) ;
#6968=CARTESIAN_POINT ( 'NONE',  ( -4.432034252711344102, 28.15327818181735964, -79.99999999999995737 ) ) ;
#6974=CIRCLE ( 'NONE', #3575, 28.50000000000000355 ) ;
#6975=DIRECTION ( 'NONE',  ( -0.9342558044690566499, -0.3566035499204627257, -1.650722232431654112E-17 ) ) ;
#6979=EDGE_CURVE ( 'NONE', #6736, #2383, #7609, .T. ) ;
#6981=VECTOR ( 'NONE', #7579, 1000.000000000000000 ) ;
#6983=CYLINDRICAL_SURFACE ( 'NONE', #7690, 29.99999999999999289 ) ;
#6984=EDGE_CURVE ( 'NONE', #7368, #6741, #5837, .T. ) ;
#6986=CARTESIAN_POINT ( 'NONE',  ( 0.000000000000000000, 0.000000000000000000, 20.00000000000000000 ) ) ;
#6988=AXIS2_PLACEMENT_3D ( 'NONE', #7436, #882, #2046 ) ;
#6993=DIRECTION ( 'NONE',  ( 0.1948910352220799280, -0.9808248999643441879, -1.110223024625155793E-18 ) ) ;
#6998=CARTESIAN_POINT ( 'NONE',  ( 10.00000000000000000, 0.000000000000000000, -50.00000000000000000 ) ) ;
#7000=LINE ( 'NONE', #1596, #600 ) ;
#7009=DIRECTION ( 'NONE',  ( 1.000000000000000000, 0.000000000000000000, 0.000000000000000000 ) ) ;
#7010=CARTESIAN_POINT ( 'NONE',  ( -6.873268260756527152E-15, 0.000000000000000000, -79.99999999999995737 ) ) ;
#7014=EDGE_CURVE ( 'NONE', #322, #3277, #68, .T. ) ;
#7029=DIRECTION ( 'NONE',  ( 0.3566035499204626702, -0.9342558044690565389, 2.649161120199466423E-17 ) ) ;
#7031=DIRECTION ( 'NONE',  ( -0.3189555096957539804, 0.9477696887085605981, -2.581026109104742702E-17 ) ) ;
#7036=DIRECTION ( 'NONE',  ( 0.000000000000000000, 0.000000000000000000, 1.000000000000000000 ) ) ;
#7039=DIRECTION ( 'NONE',  ( 0.000000000000000000, 0.000000000000000000, 1.000000000000000000 ) ) ;
#7045=ORIENTED_EDGE ( 'NONE', *, *, #3978, .T. ) ;
#7057=CARTESIAN_POINT ( 'NONE',  ( 9.090232026328989079, -27.01143612819398143, -122.9999999999999716 ) ) ;
#7063=CARTESIAN_POINT ( 'NONE',  ( -6.873268260756527152E-15, 0.000000000000000000, -79.99999999999995737 ) ) ;
#7064=DIRECTION ( 'NONE',  ( 5.551115123125782702E-17, -0.000000000000000000, 1.000000000000000000 ) ) ;
#7067=CARTESIAN_POINT ( 'NONE',  ( 2.718977167127996530, 29.87653198021210699, -139.9999999999999716 ) ) ;
#7081=EDGE_LOOP ( 'NONE', ( #264, #5557, #2606, #1267 ) ) ;
#7083=VECTOR ( 'NONE', #481, 1000.000000000000000 ) ;
#7085=CARTESIAN_POINT ( 'NONE',  ( 10.69810649761388177, -28.02767413407170238, -139.9999999999999716 ) ) ;
#7088=FACE_OUTER_BOUND ( 'NONE', #1482, .T. ) ;
#7105=AXIS2_PLACEMENT_3D ( 'NONE', #2033, #2811, #4427 ) ;
#7107=LINE ( 'NONE', #7067, #7083 ) ;
#7112=DIRECTION ( 'NONE',  ( -1.000000000000000000, 0.000000000000000000, 0.000000000000000000 ) ) ;
#7113=DIRECTION ( 'NONE',  ( 0.000000000000000000, 0.000000000000000000, -1.000000000000000000 ) ) ;
#7118=CARTESIAN_POINT ( 'NONE',  ( -10.00000000000000000, 41.99999999999999289, -60.00000000000000711 ) ) ;
#7123=ORIENTED_EDGE ( 'NONE', *, *, #1522, .F. ) ;
#7138=LINE ( 'NONE', #4650, #140 ) ;
#7142=ORIENTED_EDGE ( 'NONE', *, *, #5198, .T. ) ;
#7147=CARTESIAN_POINT ( 'NONE',  ( 0.000000000000000000, 0.000000000000000000, -119.9999999999999716 ) ) ;
#7155=DIRECTION ( 'NONE',  ( -0.9914631140645256968, 0.1303874742813643794, 0.000000000000000000 ) ) ;
#7157=DIRECTION ( 'NONE',  ( -1.000000000000000000, 0.000000000000000000, 0.000000000000000000 ) ) ;
#7160=VERTEX_POINT ( 'NONE', #4785 ) ;
#7161=ORIENTED_EDGE ( 'NONE', *, *, #573, .T. ) ;
#7165=CIRCLE ( 'NONE', #484, 35.00000000000000711 ) ;
#7166=LINE ( 'NONE', #4318, #2885 ) ;
#7167=DIRECTION ( 'NONE',  ( 0.9938725510941108787, -0.1105321318969463978, 0.000000000000000000 ) ) ;
#7169=APPLICATION_CONTEXT ( 'automotive_design' ) ;
#7186=CIRCLE ( 'NONE', #1507, 30.00000000000000355 ) ;
#7193=EDGE_LOOP ( 'NONE', ( #6905, #6155 ) ) ;
#7203=ORIENTED_EDGE ( 'NONE', *, *, #6939, .T. ) ;
#7227=DIRECTION ( 'NONE',  ( 0.000000000000000000, 0.000000000000000000, 1.000000000000000000 ) ) ;
#7237=FACE_OUTER_BOUND ( 'NONE', #1363, .T. ) ;
#7238=FACE_OUTER_BOUND ( 'NONE', #7763, .T. ) ;
#7242=ORIENTED_EDGE ( 'NONE', *, *, #6395, .T. ) ;
#7257=CARTESIAN_POINT ( 'NONE',  ( -5.846731056662405557, 29.42474699893032053, -79.99999999999995737 ) ) ;
#7259=LINE ( 'NONE', #4370, #1049 ) ;
#7261=ORIENTED_EDGE ( 'NONE', *, *, #4183, .F. ) ;
#7263=ADVANCED_FACE ( 'NONE', ( #7237 ), #7592, .F. ) ;
#7268=ORIENTED_EDGE ( 'NONE', *, *, #1084, .T. ) ;
#7276=CARTESIAN_POINT ( 'NONE',  ( 3.716043017018883621, 28.25669875083898930, 10.00000000000000000 ) ) ;
#7296=DIRECTION ( 'NONE',  ( 0.9412010056177179118, 0.3378471059875997051, 0.000000000000000000 ) ) ;
#7306=CARTESIAN_POINT ( 'NONE',  ( -10.00000000000000000, 33.54101966249685773, -50.00000000000000000 ) ) ;
#7308=ORIENTED_EDGE ( 'NONE', *, *, #5237, .T. ) ;
#7317=EDGE_CURVE ( 'NONE', #4191, #6073, #4953, .T. ) ;
#7320=VERTEX_POINT ( 'NONE', #3137 ) ;
#7324=ADVANCED_FACE ( 'NONE', ( #6090 ), #3098, .T. ) ;
#7333=ORIENTED_EDGE ( 'NONE', *, *, #5631, .T. ) ;
#7339=ORIENTED_EDGE ( 'NONE', *, *, #512, .F. ) ;
#7343=DIRECTION ( 'NONE',  ( 0.1303874742813643517, 0.9914631140645255858, 0.000000000000000000 ) ) ;
#7347=ORIENTED_EDGE ( 'NONE', *, *, #1968, .F. ) ;
#7349=CARTESIAN_POINT ( 'NONE',  ( 2.583028308771596837, 28.38270538120150377, 10.00000000000000000 ) ) ;
#7351=CARTESIAN_POINT ( 'NONE',  ( 0.000000000000000000, 0.000000000000000000, -50.00000000000000000 ) ) ;
#7357=EDGE_CURVE ( 'NONE', #3615, #6864, #3711, .T. ) ;
#7368=VERTEX_POINT ( 'NONE', #683 ) ;
#7371=ORIENTED_EDGE ( 'NONE', *, *, #7412, .T. ) ;
#7374=DIRECTION ( 'NONE',  ( 5.551115123125782702E-17, 0.000000000000000000, 1.000000000000000000 ) ) ;
#7385=CARTESIAN_POINT ( 'NONE',  ( 0.000000000000000000, 0.000000000000000000, -50.00000000000000000 ) ) ;
#7407=CIRCLE ( 'NONE', #5520, 29.99999999999999289 ) ;
#7412=EDGE_CURVE ( 'NONE', #2088, #3277, #4861, .T. ) ;
#7436=CARTESIAN_POINT ( 'NONE',  ( 0.000000000000000000, 0.000000000000000000, -139.9999999999999716 ) ) ;
#7447=VERTEX_POINT ( 'NONE', #948 ) ;
#7454=EDGE_CURVE ( 'NONE', #1043, #3634, #5213, .T. ) ;
#7455=CYLINDRICAL_SURFACE ( 'NONE', #5405, 28.50000000000000355 ) ;
#7456=CARTESIAN_POINT ( 'NONE',  ( 9.090232026328989079, -27.01143612819398143, -122.9999999999999716 ) ) ;
#7457=ORIENTED_EDGE ( 'NONE', *, *, #7317, .F. ) ;
#7458=CIRCLE ( 'NONE', #2678, 30.00000000000000355 ) ;
#7461=CARTESIAN_POINT ( 'NONE',  ( 0.000000000000000000, 0.000000000000000000, 10.00000000000000000 ) ) ;
#7470=CARTESIAN_POINT ( 'NONE',  ( -4.432034252711344102, 28.15327818181735964, -82.99999999999995737 ) ) ;
#7476=EDGE_LOOP ( 'NONE', ( #4375, #3574, #6938, #3405 ) ) ;
#7485=AXIS2_PLACEMENT_3D ( 'NONE', #1301, #3758, #5977 ) ;
#7490=FACE_OUTER_BOUND ( 'NONE', #7081, .T. ) ;
#7492=VERTEX_POINT ( 'NONE', #1505 ) ;
#7497=DIRECTION ( 'NONE',  ( 0.9412010056177179118, 0.3378471059875997051, 0.000000000000000000 ) ) ;
#7500=ORIENTED_EDGE ( 'NONE', *, *, #4379, .F. ) ;
#7503=DIRECTION ( 'NONE',  ( 3.081487911019577365E-33, -2.775557561562891967E-17, -1.000000000000000000 ) ) ;
#7509=FACE_OUTER_BOUND ( 'NONE', #6751, .T. ) ;
#7513=ADVANCED_FACE ( 'NONE', ( #3248, #6246 ), #4540, .T. ) ;
#7514=AXIS2_PLACEMENT_3D ( 'NONE', #2743, #6255, #3888 ) ;
#7520=AXIS2_PLACEMENT_3D ( 'NONE', #3877, #2661, #7497 ) ;
#7526=CARTESIAN_POINT ( 'NONE',  ( 0.000000000000000000, 0.000000000000000000, 20.00000000000000000 ) ) ;
#7530=ORIENTED_EDGE ( 'NONE', *, *, #1968, .T. ) ;
#7531=AXIS2_PLACEMENT_3D ( 'NONE', #479, #5291, #2932 ) ;
#7543=AXIS2_PLACEMENT_3D ( 'NONE', #458, #5947, #7756 ) ;
#7545=LINE ( 'NONE', #5221, #1559 ) ;
#7550=DIRECTION ( 'NONE',  ( 0.9412010056177179118, 0.3378471059875997051, 0.000000000000000000 ) ) ;
#7565=ORIENTED_EDGE ( 'NONE', *, *, #1377, .T. ) ;
#7570=ORIENTED_EDGE ( 'NONE', *, *, #5964, .F. ) ;
#7579=DIRECTION ( 'NONE',  ( 0.000000000000000000, 1.000000000000000000, 0.000000000000000000 ) ) ;
#7586=ORIENTED_EDGE ( 'NONE', *, *, #48, .F. ) ;
#7588=ADVANCED_FACE ( 'NONE', ( #3445 ), #3294, .T. ) ;
#7592=PLANE ( 'NONE',  #916 ) ;
#7593=CARTESIAN_POINT ( 'NONE',  ( 29.99999999999999289, 0.000000000000000000, -79.99999999999995737 ) ) ;
#7594=DIRECTION ( 'NONE',  ( 0.000000000000000000, 0.000000000000000000, 1.000000000000000000 ) ) ;
#7603=VERTEX_POINT ( 'NONE', #3919 ) ;
#7609=LINE ( 'NONE', #4021, #6718 ) ;
#7613=FACE_OUTER_BOUND ( 'NONE', #292, .T. ) ;
#7626=CARTESIAN_POINT ( 'NONE',  ( -1.728922298134113098E-15, 8.513302795252935035E-16, 13.00000000000000178 ) ) ;
#7642=VERTEX_POINT ( 'NONE', #1552 ) ;
#7643=DIRECTION ( 'NONE',  ( 0.000000000000000000, 0.000000000000000000, 1.000000000000000000 ) ) ;
#7644=EDGE_CURVE ( 'NONE', #1102, #6819, #5692, .T. ) ;
#7653=CARTESIAN_POINT ( 'NONE',  ( 0.000000000000000000, 0.000000000000000000, -50.00000000000000000 ) ) ;
#7654=LINE ( 'NONE', #6403, #4889 ) ;
#7655=VECTOR ( 'NONE', #6757, 1000.000000000000000 ) ;
#7658=ORIENTED_EDGE ( 'NONE', *, *, #2357, .T. ) ;
#7679=ORIENTED_EDGE ( 'NONE', *, *, #7644, .F. ) ;
#7685=SURFACE_STYLE_USAGE ( .BOTH. , #1059 ) ;
#7687=CARTESIAN_POINT ( 'NONE',  ( -26.82422866010496776, -9.628642520646595315, -122.9999999999999716 ) ) ;
#7690=AXIS2_PLACEMENT_3D ( 'NONE', #267, #5081, #2104 ) ;
#7693=EDGE_CURVE ( 'NONE', #7603, #1043, #6292, .T. ) ;
#7695=CYLINDRICAL_SURFACE ( 'NONE', #3284, 28.50000000000000355 ) ;
#7698=CARTESIAN_POINT ( 'NONE',  ( 0.000000000000000000, 0.000000000000000000, 20.00000000000000000 ) ) ;
#7701=EDGE_CURVE ( 'NONE', #2888, #5846, #7545, .T. ) ;
#7711=FACE_OUTER_BOUND ( 'NONE', #775, .T. ) ;
#7728=DIRECTION ( 'NONE',  ( 0.9845265360683707057, 0.1752355551171480841, 0.000000000000000000 ) ) ;
#7737=( GEOMETRIC_REPRESENTATION_CONTEXT ( 3 ) GLOBAL_UNCERTAINTY_ASSIGNED_CONTEXT ( ( #4881 ) ) GLOBAL_UNIT_ASSIGNED_CONTEXT ( ( #5796, #1016, #6466 ) ) REPRESENTATION_CONTEXT ( 'NONE', 'WORKASPACE' ) );
#7746=CARTESIAN_POINT ( 'NONE',  ( 0.000000000000000000, 0.000000000000000000, -82.99999999999995737 ) ) ;
#7756=DIRECTION ( 'NONE',  ( 0.9845265360683707057, 0.1752355551171480841, 0.000000000000000000 ) ) ;
#7757=ADVANCED_FACE ( 'NONE', ( #526 ), #4300, .F. ) ;
#7760=VECTOR ( 'NONE', #2549, 1000.000000000000114 ) ;
#7763=EDGE_LOOP ( 'NONE', ( #3339, #1627, #1383, #7457, #6582, #2052, #5896, #1495 ) ) ;
#7824=COLOUR_RGB('Grey',0.48,0.52,0.57);
#7825=FILL_AREA_STYLE_COLOUR('',#7824);
#7826=FILL_AREA_STYLE('',(#7825));
#7827=SURFACE_STYLE_FILL_AREA(#7826);
#7828=SURFACE_SIDE_STYLE('',(#7827));
#7829=SURFACE_STYLE_USAGE(.BOTH.,#7828);
#7830=PRESENTATION_STYLE_ASSIGNMENT((#7829));
ENDSEC;
END-ISO-10303-21;
